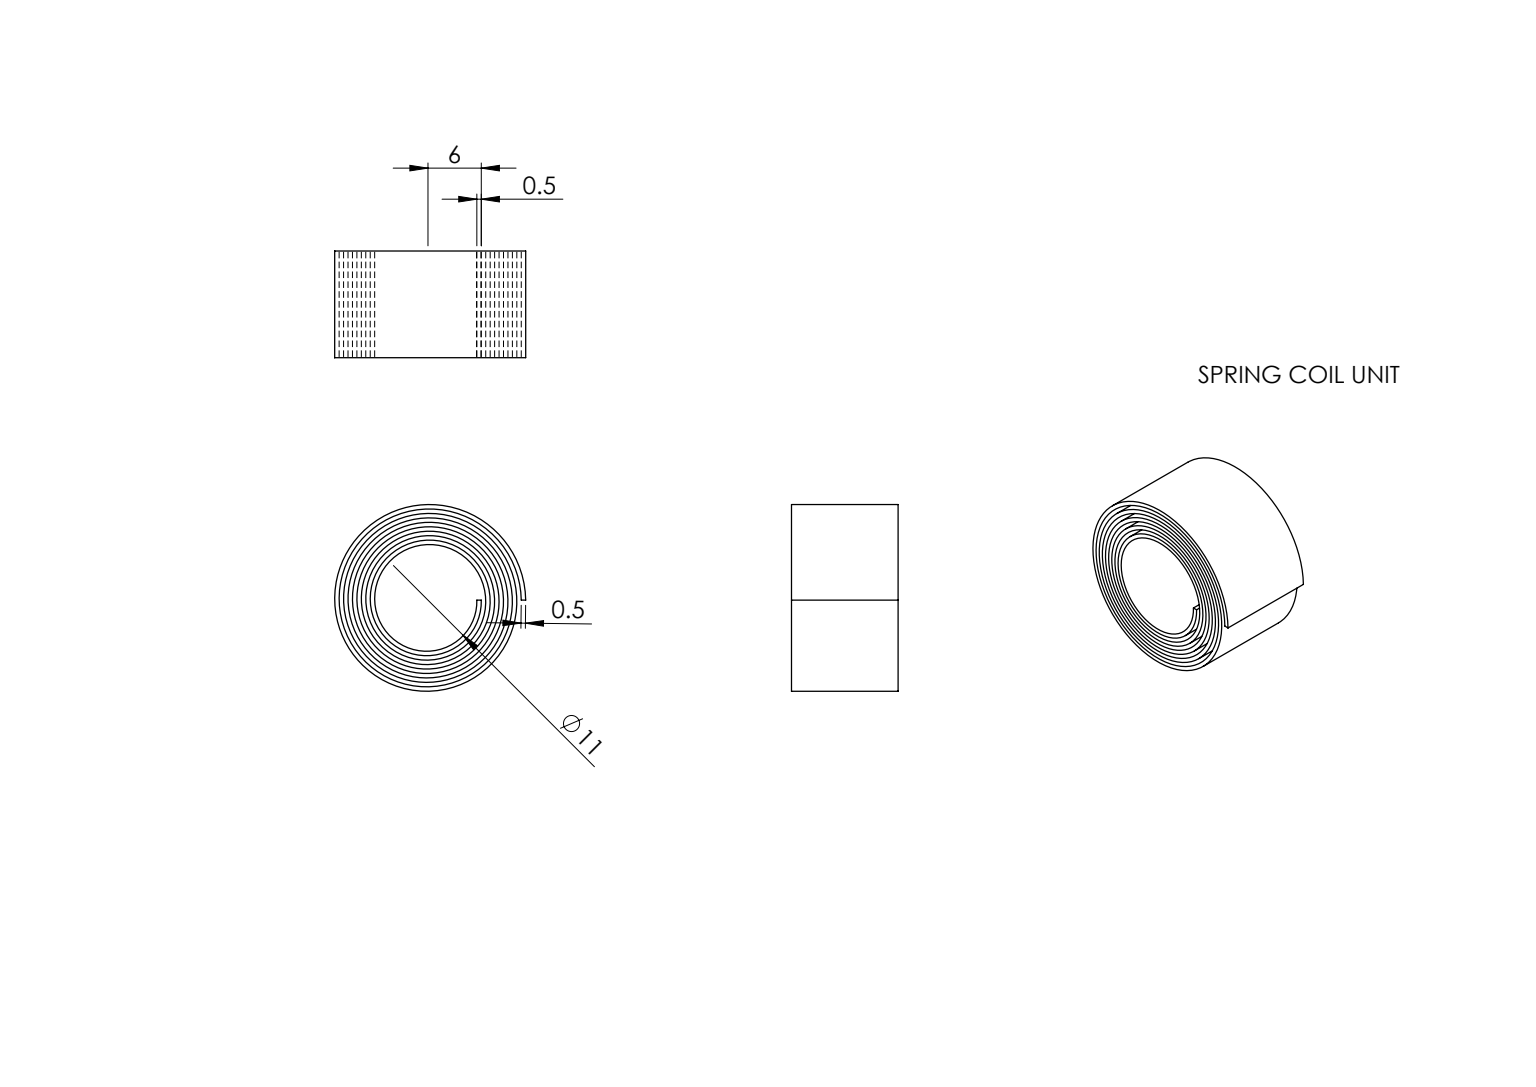
ISO-10303-21;
HEADER;
FILE_DESCRIPTION (('STEP AP214'),
    '1' );
FILE_NAME ('Spring Coil Unit.step',
    '2026-10-23T14:45:25',
    ( '' ),
    ( '' ),
    'SwSTEP 2.0',
    'SolidWorks 2026',
    '' );
FILE_SCHEMA (( 'AUTOMOTIVE_DESIGN' ));
ENDSEC;

DATA;
#1=CARTESIAN_POINT ( 'NONE',  ( -5.525185448606692695, 2.707100724334796649, 1.999999999999998224 ) ) ;
#7=CARTESIAN_POINT ( 'NONE',  ( 10.06493078320225010, 4.366638945734137245, 13.99999999999999645 ) ) ;
#13=CARTESIAN_POINT ( 'NONE',  ( 8.453438707197836521, 0.9797652757261499090, 14.00000000000000000 ) ) ;
#14=CARTESIAN_POINT ( 'NONE',  ( 3.892125705850321804, -6.036954802193386982, 1.999999999999998224 ) ) ;
#16=CARTESIAN_POINT ( 'NONE',  ( 7.990059919442007441, -3.149571442993018167, 14.00000000000000000 ) ) ;
#18=CARTESIAN_POINT ( 'NONE',  ( -2.440069559021881496, 10.46881825416662259, 1.999999999999998224 ) ) ;
#20=CARTESIAN_POINT ( 'NONE',  ( 5.887534416617372202, 3.663839002572494952, 13.99999999999999645 ) ) ;
#22=CARTESIAN_POINT ( 'NONE',  ( -2.415560149437878668, -8.486491385245608754, 1.999999999999998224 ) ) ;
#24=CARTESIAN_POINT ( 'NONE',  ( 2.877506500681688006, 7.288437455188073955, 1.999999999999998224 ) ) ;
#32=CARTESIAN_POINT ( 'NONE',  ( -10.48421140591525713, 1.206973991593908169, 13.99999999999999645 ) ) ;
#33=AXIS2_PLACEMENT_3D ( 'NONE', #3461, #5223, #4408 ) ;
#38=CARTESIAN_POINT ( 'NONE',  ( -0.2798806129217078498, -8.779921314117062892, 14.00000000000000000 ) ) ;
#39=CARTESIAN_POINT ( 'NONE',  ( 6.444084565535371567, 4.617298776321547393, 1.999999999999998224 ) ) ;
#42=CARTESIAN_POINT ( 'NONE',  ( -2.415560149437796511, -8.486491385245610530, 14.00000000000000000 ) ) ;
#45=CARTESIAN_POINT ( 'NONE',  ( 8.595497693523489247, -5.345940745659027549, 1.999999999999998224 ) ) ;
#46=CARTESIAN_POINT ( 'NONE',  ( -5.651290410005069376, 9.082320918485367045, 1.999999999999998224 ) ) ;
#47=( GEOMETRIC_REPRESENTATION_CONTEXT ( 3 ) GLOBAL_UNCERTAINTY_ASSIGNED_CONTEXT ( ( #114 ) ) GLOBAL_UNIT_ASSIGNED_CONTEXT ( ( #3594, #2760, #4052 ) ) REPRESENTATION_CONTEXT ( 'NONE', 'WORKASPACE' ) );
#48=CARTESIAN_POINT ( 'NONE',  ( -1.424809953814591523, 6.586142414399822620, 13.99999999999999645 ) ) ;
#49=CARTESIAN_POINT ( 'NONE',  ( 7.716263785693136867, -3.801003699432787375, 1.999999999999998224 ) ) ;
#51=CARTESIAN_POINT ( 'NONE',  ( 6.638644669766898154, 2.135480210976827387, 1.999999999999998224 ) ) ;
#61=CARTESIAN_POINT ( 'NONE',  ( -3.798941939731700579, -9.621416145859109648, 13.99999999999999645 ) ) ;
#66=CARTESIAN_POINT ( 'NONE',  ( -7.161907081466633684, 5.673982509929174967, 14.00000000000000000 ) ) ;
#67=CARTESIAN_POINT ( 'NONE',  ( 7.024953159363688471, -4.052930060063556716, 1.999999999999998224 ) ) ;
#70=CARTESIAN_POINT ( 'NONE',  ( -7.550296695603107899, -2.566425989403007257, 1.999999999999998224 ) ) ;
#71=CARTESIAN_POINT ( 'NONE',  ( 0.7514524083000287957, 9.263466152293682754, 14.00000000000000000 ) ) ;
#74=CARTESIAN_POINT ( 'NONE',  ( 9.807503887220748950, -2.283819133639664489, 1.999999999999998224 ) ) ;
#75=CARTESIAN_POINT ( 'NONE',  ( 6.160418207306094018, 1.983851483784787373, 14.00000000000000000 ) ) ;
#76=CARTESIAN_POINT ( 'NONE',  ( -7.091148812992124739, -4.571561645351811976, 13.99999999999999645 ) ) ;
#77=CARTESIAN_POINT ( 'NONE',  ( -8.026550172065741506, -2.724140490265046122, 13.99999999999999645 ) ) ;
#79=CARTESIAN_POINT ( 'NONE',  ( -4.424777426321968576, -7.679192617323552739, 1.999999999999998224 ) ) ;
#80=CARTESIAN_POINT ( 'NONE',  ( 5.887534416617370425, 3.663839002572738313, 1.999999999999998224 ) ) ;
#89=CARTESIAN_POINT ( 'NONE',  ( -8.483256258862985177, -6.077987531410205868, 13.99999999999999645 ) ) ;
#95=CARTESIAN_POINT ( 'NONE',  ( -6.708753103182797162, 7.642576097240647570, 14.00000000000000000 ) ) ;
#96=CARTESIAN_POINT ( 'NONE',  ( 7.409328306158467825, 2.927536720054290775, 1.999999999999998224 ) ) ;
#97=CARTESIAN_POINT ( 'NONE',  ( 5.612687125617794592, -6.603876269260512188, 1.999999999999998224 ) ) ;
#98=CARTESIAN_POINT ( 'NONE',  ( -6.185289998984974780, -6.402116997106622520, 14.00000000000000000 ) ) ;
#100=CARTESIAN_POINT ( 'NONE',  ( -0.7077576507783156501, 10.75210906117156995, 1.999999999999998224 ) ) ;
#102=CARTESIAN_POINT ( 'NONE',  ( 5.103689747953259470, 6.014827819656690444, 13.99999999999999645 ) ) ;
#103=CARTESIAN_POINT ( 'NONE',  ( -8.388197440585694054, -1.387539741535495974, 13.99999999999999645 ) ) ;
#104=CARTESIAN_POINT ( 'NONE',  ( 1.492118473828444536, -5.588909376072072277, 14.00000000000000000 ) ) ;
#106=CARTESIAN_POINT ( 'NONE',  ( -8.126042061586874254, 2.755650963504471473, 1.999999999999998224 ) ) ;
#108=CARTESIAN_POINT ( 'NONE',  ( -0.5497243705170606898, -6.763214047005217999, 1.999999999999998224 ) ) ;
#113=SURFACE_STYLE_FILL_AREA ( #890 ) ;
#114=UNCERTAINTY_MEASURE_WITH_UNIT (LENGTH_MEASURE( 1.000000000000000082E-05 ), #3594, 'distance_accuracy_value', 'NONE');
#115=CARTESIAN_POINT ( 'NONE',  ( 5.800093669798302543, -8.375184749302979625, 13.99999999999999645 ) ) ;
#119=CARTESIAN_POINT ( 'NONE',  ( -3.139313036748870189, 9.741172307225710369, 14.00000000000000000 ) ) ;
#120=CARTESIAN_POINT ( 'NONE',  ( -0.2539011084975961174, 7.766605221862830533, 1.999999999999998224 ) ) ;
#122=CARTESIAN_POINT ( 'NONE',  ( -8.763921109942213405, 2.343993041296470459, 1.999999999999998224 ) ) ;
#123=CARTESIAN_POINT ( 'NONE',  ( -7.559400777704423646, -6.425066744314204215, 14.00000000000000000 ) ) ;
#126=CARTESIAN_POINT ( 'NONE',  ( 7.631804465921431913, -6.689046765414639495, 1.999999999999998224 ) ) ;
#129=CARTESIAN_POINT ( 'NONE',  ( 0.5754137710878940437, 8.770917875152660415, 13.99999999999999645 ) ) ;
#131=CARTESIAN_POINT ( 'NONE',  ( -9.772156678340820690, -2.119544458102139206, 1.999999999999998224 ) ) ;
#133=CARTESIAN_POINT ( 'NONE',  ( 3.747087600548639763, -7.295897990121164689, 1.999999999999998224 ) ) ;
#137=CARTESIAN_POINT ( 'NONE',  ( -7.019651866617071079, -0.1200674265790944856, 1.999999999999998224 ) ) ;
#140=CARTESIAN_POINT ( 'NONE',  ( -3.597458971453999066, 6.226096630968013024, 1.999999999999998224 ) ) ;
#152=CARTESIAN_POINT ( 'NONE',  ( -9.772156678340820690, -2.119544458102511353, 14.00000000000000000 ) ) ;
#153=CARTESIAN_POINT ( 'NONE',  ( 7.344045208304290639, 5.086154276871864610, 1.999999999999998224 ) ) ;
#156=CARTESIAN_POINT ( 'NONE',  ( 4.415008247871750058, 7.106745273741266189, 1.999999999999998224 ) ) ;
#157=CARTESIAN_POINT ( 'NONE',  ( -4.983290658054754019, 7.721050520723660604, 14.00000000000000000 ) ) ;
#162=CARTESIAN_POINT ( 'NONE',  ( -5.390757458300978300, 6.793134358447313836, 13.99999999999999645 ) ) ;
#164=CARTESIAN_POINT ( 'NONE',  ( -0.6809175113353352904, 10.25113960786383771, 1.999999999999998224 ) ) ;
#166=CARTESIAN_POINT ( 'NONE',  ( 3.388254439433305176, -8.575817650944026482, 1.999999999999998224 ) ) ;
#170=CARTESIAN_POINT ( 'NONE',  ( -1.320393794063943416, 6.095439640211752774, 1.999999999999998224 ) ) ;
#172=CARTESIAN_POINT ( 'NONE',  ( -4.975175822334872322, 5.137265612443480123, 1.999999999999998224 ) ) ;
#178=LINE ( 'NONE', #3662, #4829 ) ;
#181=CARTESIAN_POINT ( 'NONE',  ( 0.7514524083000287957, 9.263466152293682754, 14.00000000000000000 ) ) ;
#182=CARTESIAN_POINT ( 'NONE',  ( 4.043470907200509501, 7.877814422643418801, 1.999999999999998224 ) ) ;
#183=CARTESIAN_POINT ( 'NONE',  ( -1.480145937554574020, 8.115026467928048604, 1.999999999999998224 ) ) ;
#184=CARTESIAN_POINT ( 'NONE',  ( 7.258279873954945671, -6.354128476750924293, 14.00000000000000000 ) ) ;
#188=CARTESIAN_POINT ( 'NONE',  ( 5.326024957120313985, -1.813589758486611858, 14.00000000000000000 ) ) ;
#189=CARTESIAN_POINT ( 'NONE',  ( -2.179108132477381332, -10.08557389312607278, 13.99999999999999645 ) ) ;
#191=CARTESIAN_POINT ( 'NONE',  ( 3.896371052708265559, -4.167854722423870228, 14.00000000000000000 ) ) ;
#193=CARTESIAN_POINT ( 'NONE',  ( -1.063411474431080306, -9.238278818534249481, 1.999999999999998224 ) ) ;
#195=CARTESIAN_POINT ( 'NONE',  ( -6.742266116715657454, -1.811900715329134215, 1.999999999999998224 ) ) ;
#197=ORIENTED_EDGE ( 'NONE', *, *, #3580, .T. ) ;
#198=CARTESIAN_POINT ( 'NONE',  ( -6.041022033915842471, 3.753782041846908779, 1.999999999999998224 ) ) ;
#200=CARTESIAN_POINT ( 'NONE',  ( -3.379911625893651017, -5.460782782531100388, 13.99999999999999645 ) ) ;
#208=CARTESIAN_POINT ( 'NONE',  ( -8.440272934376206848, 1.393994921405934173, 1.999999999999998224 ) ) ;
#209=CARTESIAN_POINT ( 'NONE',  ( 4.326322805050086373, -6.952463250691143237, 13.99999999999999645 ) ) ;
#210=CARTESIAN_POINT ( 'NONE',  ( -2.067895747887561697, -9.596367745172036834, 1.999999999999998224 ) ) ;
#216=CARTESIAN_POINT ( 'NONE',  ( -1.105557477332586691, -6.708264047591377732, 14.00000000000000000 ) ) ;
#217=CARTESIAN_POINT ( 'NONE',  ( -8.745075223331019387, 3.959260399367729111, 13.99999999999999645 ) ) ;
#218=CARTESIAN_POINT ( 'NONE',  ( -4.354965481614496703, -8.841480220787186539, 1.999999999999998224 ) ) ;
#221=CARTESIAN_POINT ( 'NONE',  ( -0.1359230501497094012, -8.279147739300480424, 1.999999999999998224 ) ) ;
#226=CARTESIAN_POINT ( 'NONE',  ( 2.227988792049259814, 5.923272706911028251, 1.999999999999998224 ) ) ;
#228=CARTESIAN_POINT ( 'NONE',  ( 3.520917041835318173, -6.848083076130971669, 1.999999999999998224 ) ) ;
#236=CARTESIAN_POINT ( 'NONE',  ( -0.1359230501497094012, -8.279147739300480424, 1.999999999999998224 ) ) ;
#237=CARTESIAN_POINT ( 'NONE',  ( -5.921118896519415919, 6.318058289644736369, 13.99999999999999645 ) ) ;
#243=CARTESIAN_POINT ( 'NONE',  ( 6.004028658818958419, -2.715480180205860794, 14.00000000000000000 ) ) ;
#244=CARTESIAN_POINT ( 'NONE',  ( 3.917689075872249571, 9.035181080458080771, 13.99999999999999645 ) ) ;
#245=CARTESIAN_POINT ( 'NONE',  ( -0.5497243705170608008, -6.763214047005219776, 14.00000000000000000 ) ) ;
#249=CARTESIAN_POINT ( 'NONE',  ( -10.48421140591450751, 1.206973991593908169, 1.999999999999998224 ) ) ;
#253=CARTESIAN_POINT ( 'NONE',  ( 6.680730669075649608, 3.301097878975988387, 1.999999999999998224 ) ) ;
#255=CARTESIAN_POINT ( 'NONE',  ( -5.416162817796314144, -4.301262981183148426, 1.999999999999998224 ) ) ;
#256=CARTESIAN_POINT ( 'NONE',  ( -2.466819000628106551, 6.242838961510105200, 1.999999999999998224 ) ) ;
#258=CARTESIAN_POINT ( 'NONE',  ( 4.793600759081160234, 4.956424179878266223, 13.99999999999999645 ) ) ;
#261=VERTEX_POINT ( 'NONE', #4126 ) ;
#264=CARTESIAN_POINT ( 'NONE',  ( 3.747087600548639763, -7.295897990121164689, 1.999999999999998224 ) ) ;
#265=CARTESIAN_POINT ( 'NONE',  ( -7.364573508975984062, 1.714675912027187943, 13.99999999999999645 ) ) ;
#266=CARTESIAN_POINT ( 'NONE',  ( 5.030817567586885808, 9.062633982223131213, 14.00000000000000000 ) ) ;
#269=PRODUCT_DEFINITION_SHAPE ( 'NONE', 'NONE',  #3907 ) ;
#273=CARTESIAN_POINT ( 'NONE',  ( -2.717942380035140992, -6.274577315194989957, 14.00000000000000000 ) ) ;
#274=CARTESIAN_POINT ( 'NONE',  ( -1.592064345877354903, 9.625584969239746158, 13.99999999999999645 ) ) ;
#275=CARTESIAN_POINT ( 'NONE',  ( 4.290186206382709422, 5.996800006796702220, 14.00000000000000000 ) ) ;
#277=CARTESIAN_POINT ( 'NONE',  ( 7.631804465921431913, -6.689046765414639495, 1.999999999999998224 ) ) ;
#280=CARTESIAN_POINT ( 'NONE',  ( -7.652305818843809782, 2.590529227167489790, 1.999999999999998224 ) ) ;
#282=CARTESIAN_POINT ( 'NONE',  ( -1.189470317277863565, -7.202885406307538041, 13.99999999999999645 ) ) ;
#283=CARTESIAN_POINT ( 'NONE',  ( 0.000000000000000000, 0.000000000000000000, 0.000000000000000000 ) ) ;
#289=CARTESIAN_POINT ( 'NONE',  ( -8.017392084630253990, -4.988806607527433989, 1.999999999999998224 ) ) ;
#290=CARTESIAN_POINT ( 'NONE',  ( 8.697835924490034287, 4.836984431370582982, 13.99999999999999645 ) ) ;
#291=CARTESIAN_POINT ( 'NONE',  ( 9.925004466819306259, 3.374327561486830440, 14.00000000000000000 ) ) ;
#296=CARTESIAN_POINT ( 'NONE',  ( -5.034899347480884302, -4.722558430572732391, 14.00000000000000000 ) ) ;
#297=CARTESIAN_POINT ( 'NONE',  ( 5.099673838353210975, -8.834479793763010846, 13.99999999999999645 ) ) ;
#299=CARTESIAN_POINT ( 'NONE',  ( 7.439669587982604249, 0.9822684312230363091, 14.00000000000000000 ) ) ;
#301=CARTESIAN_POINT ( 'NONE',  ( -8.017392084630253990, -4.988806607527433989, 1.999999999999998224 ) ) ;
#305=CARTESIAN_POINT ( 'NONE',  ( 6.929006764466009827, 4.804313515625705300, 1.999999999999998224 ) ) ;
#307=CARTESIAN_POINT ( 'NONE',  ( 4.243312049792013596, -4.537448458213932945, 1.999999999999998224 ) ) ;
#308=CARTESIAN_POINT ( 'NONE',  ( -7.375360291558942905, -1.341686286798741357, 13.99999999999999645 ) ) ;
#311=CARTESIAN_POINT ( 'NONE',  ( -4.354965481614496703, -8.841480220787186539, 1.999999999999998224 ) ) ;
#320=CARTESIAN_POINT ( 'NONE',  ( 6.971023843911450690, -5.915260676233724091, 13.99999999999999645 ) ) ;
#321=CARTESIAN_POINT ( 'NONE',  ( 8.774740126074163982, 5.663528079765788981, 14.00000000000000000 ) ) ;
#327=CARTESIAN_POINT ( 'NONE',  ( -6.334648143026945455, -2.872559841354017429, 14.00000000000000000 ) ) ;
#329=CARTESIAN_POINT ( 'NONE',  ( 10.40193138080327628, 3.529992181067589829, 13.99999999999999645 ) ) ;
#332=CARTESIAN_POINT ( 'NONE',  ( 4.443413384189735638, 4.597174039215665253, 14.00000000000000000 ) ) ;
#335=CARTESIAN_POINT ( 'NONE',  ( 9.807503887220748950, -2.283819133639664489, 1.999999999999998224 ) ) ;
#339=CARTESIAN_POINT ( 'NONE',  ( 6.037635170864973588, 5.848285684830694997, 1.999999999999998224 ) ) ;
#343=CARTESIAN_POINT ( 'NONE',  ( 6.997680802075244344, 0.4609939245309428446, 13.99999999999999645 ) ) ;
#344=CARTESIAN_POINT ( 'NONE',  ( -9.772156678340820690, -2.119544458102139206, 1.999999999999998224 ) ) ;
#351=CARTESIAN_POINT ( 'NONE',  ( 2.701324588234351953, 8.405562337868641265, 13.99999999999999645 ) ) ;
#358=CARTESIAN_POINT ( 'NONE',  ( 8.156937663706065322, 2.333191796391004047, 14.00000000000000000 ) ) ;
#359=CARTESIAN_POINT ( 'NONE',  ( -7.945634105012030268, -6.745245841439798440, 13.99999999999999645 ) ) ;
#361=CARTESIAN_POINT ( 'NONE',  ( 6.523553822664519330, -0.1051741892335816969, 14.00000000000000000 ) ) ;
#363=CARTESIAN_POINT ( 'NONE',  ( -4.581738566658409617, -9.288989786611782762, 1.999999999999998224 ) ) ;
#365=CARTESIAN_POINT ( 'NONE',  ( -5.623512120026317618, -3.262381593763366450, 13.99999999999999645 ) ) ;
#366=CARTESIAN_POINT ( 'NONE',  ( 7.097632634466812362, -2.668286824979932970, 1.999999999999998224 ) ) ;
#368=CARTESIAN_POINT ( 'NONE',  ( 5.586635445632386343, -4.430858740432560339, 13.99999999999999645 ) ) ;
#369=CARTESIAN_POINT ( 'NONE',  ( -8.332455577110955858, 5.761155596213678010, 1.999999999999998224 ) ) ;
#375=CARTESIAN_POINT ( 'NONE',  ( -0.7976699882156008670, 9.736979168371714621, 13.99999999999999645 ) ) ;
#376=PLANE ( 'NONE',  #33 ) ;
#381=CARTESIAN_POINT ( 'NONE',  ( -7.550296695602809471, -2.566425989403007257, 14.00000000000000000 ) ) ;
#382=CARTESIAN_POINT ( 'NONE',  ( 1.869626052002579808, 6.555486721476420087, 1.999999999999998224 ) ) ;
#386=CARTESIAN_POINT ( 'NONE',  ( -6.453089103408906624, 4.947336467533685500, 14.00000000000000000 ) ) ;
#390=CARTESIAN_POINT ( 'NONE',  ( 5.213743241621229707, -4.883528188333805531, 13.99999999999999645 ) ) ;
#392=CARTESIAN_POINT ( 'NONE',  ( -8.999716648909558359, -0.5976852874978595409, 1.999999999999998224 ) ) ;
#393=CARTESIAN_POINT ( 'NONE',  ( 5.103689747953258582, 6.014827819656408892, 1.999999999999998224 ) ) ;
#394=CARTESIAN_POINT ( 'NONE',  ( 7.024953159363689359, -4.052930060063556716, 13.99999999999999645 ) ) ;
#397=( LENGTH_UNIT ( ) NAMED_UNIT ( * ) SI_UNIT ( .MILLI., .METRE. ) );
#399=CARTESIAN_POINT ( 'NONE',  ( -8.072272399572318236, -5.790267008923112080, 1.999999999999998224 ) ) ;
#406=CARTESIAN_POINT ( 'NONE',  ( 8.640499015841685448, 2.466831329604985079, 13.99999999999999645 ) ) ;
#415=CARTESIAN_POINT ( 'NONE',  ( 5.528193227149303723, 6.314447692498919018, 14.00000000000000000 ) ) ;
#416=CARTESIAN_POINT ( 'NONE',  ( -9.197478219253614640, 5.306711421960436326, 13.99999999999999645 ) ) ;
#419=CARTESIAN_POINT ( 'NONE',  ( 1.760389272475214373, -7.536528230137969686, 14.00000000000000000 ) ) ;
#423=CARTESIAN_POINT ( 'NONE',  ( -3.379911625893651017, -5.460782782531100388, 13.99999999999999645 ) ) ;
#425=CARTESIAN_POINT ( 'NONE',  ( -6.700137237869126849, -5.881230172875862472, 1.999999999999998224 ) ) ;
#427=ORIENTED_EDGE ( 'NONE', *, *, #2908, .T. ) ;
#428=CARTESIAN_POINT ( 'NONE',  ( -5.402835942920797940, -5.063607225391133504, 1.999999999999998224 ) ) ;
#439=CARTESIAN_POINT ( 'NONE',  ( -7.945634105012030268, -6.745245841439798440, 13.99999999999999645 ) ) ;
#440=ORIENTED_EDGE ( 'NONE', *, *, #5176, .T. ) ;
#444=CARTESIAN_POINT ( 'NONE',  ( -8.547479018125100581, -2.754496926847988636, 14.00000000000000000 ) ) ;
#445=CARTESIAN_POINT ( 'NONE',  ( -3.379911625893426308, -5.460782782531098611, 1.999999999999998224 ) ) ;
#448=CARTESIAN_POINT ( 'NONE',  ( 2.369394374793903246, -7.353877281245580377, 14.00000000000000000 ) ) ;
#450=CARTESIAN_POINT ( 'NONE',  ( 10.86297249782008123, 1.796588950249126349, 1.999999999999998224 ) ) ;
#451=CARTESIAN_POINT ( 'NONE',  ( 6.804422688527093754, 1.586354726854036112, 13.99999999999999645 ) ) ;
#453=CARTESIAN_POINT ( 'NONE',  ( -1.001529162299556797, -8.740421795711002417, 1.999999999999998224 ) ) ;
#454=CARTESIAN_POINT ( 'NONE',  ( 6.460119401626724489, -2.924461030940388895, 1.999999999999998224 ) ) ;
#456=SURFACE_SIDE_STYLE ('',( #113 ) ) ;
#458=CARTESIAN_POINT ( 'NONE',  ( 3.622712361020122618, 5.236663886535374957, 1.999999999999998224 ) ) ;
#462=CARTESIAN_POINT ( 'NONE',  ( -8.741731599017841248, 6.051300285686072478, 13.99999999999999645 ) ) ;
#467=CARTESIAN_POINT ( 'NONE',  ( -6.453089103408906624, 4.947336467533685500, 14.00000000000000000 ) ) ;
#468=CARTESIAN_POINT ( 'NONE',  ( 2.877506500681688006, 7.288437455188073955, 1.999999999999998224 ) ) ;
#469=DIRECTION ( 'NONE',  ( 0.000000000000000000, -0.000000000000000000, 1.000000000000000000 ) ) ;
#470=CARTESIAN_POINT ( 'NONE',  ( 7.311638624438943523, 4.225618826270838291, 14.00000000000000000 ) ) ;
#472=CARTESIAN_POINT ( 'NONE',  ( -6.726831604608804582, -7.927219868180728213, 1.999999999999998224 ) ) ;
#476=CARTESIAN_POINT ( 'NONE',  ( 3.433597602020624251, -9.098706718023301221, 1.999999999999998224 ) ) ;
#478=CARTESIAN_POINT ( 'NONE',  ( -7.227555219266156072, -1.939125212622417660, 1.999999999999998224 ) ) ;
#482=CARTESIAN_POINT ( 'NONE',  ( 2.389076732465379216, -5.237771676861643577, 1.999999999999998224 ) ) ;
#483=CARTESIAN_POINT ( 'NONE',  ( -5.021280548121167975, 3.603657539922314967, 2.000000000001176392 ) ) ;
#487=CARTESIAN_POINT ( 'NONE',  ( 2.803319092186594474, 10.45862564946370021, 13.99999999999999645 ) ) ;
#494=CARTESIAN_POINT ( 'NONE',  ( 3.713512749563263604, 8.576920285551967282, 14.00000000000000000 ) ) ;
#495=CARTESIAN_POINT ( 'NONE',  ( 7.761517335261689965, -2.213789340049559407, 1.999999999999998224 ) ) ;
#497=CARTESIAN_POINT ( 'NONE',  ( -6.453089103408601090, 4.947336467533990145, 1.999999999999998224 ) ) ;
#498=CARTESIAN_POINT ( 'NONE',  ( -3.391372024942433949, 7.476497417048839189, 14.00000000000000000 ) ) ;
#502=CARTESIAN_POINT ( 'NONE',  ( 9.077580196902394150, 4.112174628513753483, 1.999999999999998224 ) ) ;
#503=CARTESIAN_POINT ( 'NONE',  ( -2.283612537812034216, 5.775797914528924437, 14.00000000000000000 ) ) ;
#504=CARTESIAN_POINT ( 'NONE',  ( -8.026550172065741506, -2.724140490265046122, 13.99999999999999645 ) ) ;
#506=CARTESIAN_POINT ( 'NONE',  ( 2.877506500681688895, 7.288437455188075731, 13.99999999999999645 ) ) ;
#508=CARTESIAN_POINT ( 'NONE',  ( -9.031632682309719939, 0.1436733667526190195, 1.999999999999998224 ) ) ;
#510=CLOSED_SHELL ( 'NONE', ( #4640, #572, #825, #4442, #4161, #3825 ) ) ;
#511=VECTOR ( 'NONE', #2427, 1000.000000000000000 ) ;
#512=CARTESIAN_POINT ( 'NONE',  ( 7.937472058416057408, 1.044590838406009414, 1.999999999999998224 ) ) ;
#513=CARTESIAN_POINT ( 'NONE',  ( 6.000000000000000000, 0.000000000000000000, 1.999999999999998224 ) ) ;
#518=CARTESIAN_POINT ( 'NONE',  ( -3.595699629853521984, 5.016010494498948091, 1.999999999999998224 ) ) ;
#527=CARTESIAN_POINT ( 'NONE',  ( -8.765969750978372943, 5.050798838973364902, 14.00000000000000000 ) ) ;
#528=CARTESIAN_POINT ( 'NONE',  ( -0.8890388043606449742, 7.706404363472288743, 1.999999999999998224 ) ) ;
#531=CARTESIAN_POINT ( 'NONE',  ( -5.048038583874033591, -7.300734008993713609, 1.999999999999998224 ) ) ;
#532=CARTESIAN_POINT ( 'NONE',  ( -6.398096652174581678, -7.548242073784473760, 14.00000000000000000 ) ) ;
#535=CARTESIAN_POINT ( 'NONE',  ( -3.287100391418392942, 10.22059872437900019, 1.999999999999998224 ) ) ;
#536=CARTESIAN_POINT ( 'NONE',  ( 3.896371052708265559, -4.167854722423870228, 14.00000000000000000 ) ) ;
#537=CARTESIAN_POINT ( 'NONE',  ( -5.210352092881700869, -6.569156856910654874, 13.99999999999999645 ) ) ;
#538=CARTESIAN_POINT ( 'NONE',  ( 3.747087600548785868, -7.295897990121166465, 13.99999999999999645 ) ) ;
#539=CARTESIAN_POINT ( 'NONE',  ( -6.069783318623454882, -0.2142533344233820691, 14.00000000000000000 ) ) ;
#540=CARTESIAN_POINT ( 'NONE',  ( -2.153669193480073574, -8.035861145135083206, 1.999999999999998224 ) ) ;
#548=CARTESIAN_POINT ( 'NONE',  ( -5.651290410005071152, 9.082320918485368821, 13.99999999999999645 ) ) ;
#550=CARTESIAN_POINT ( 'NONE',  ( 6.000000000000000000, 0.000000000000000000, 1.999999999999998224 ) ) ;
#553=CARTESIAN_POINT ( 'NONE',  ( -5.592500163774714039, 7.275211197852027745, 14.00000000000000000 ) ) ;
#554=CARTESIAN_POINT ( 'NONE',  ( 7.025143070632193343, -0.1151745751371896220, 1.999999999999998224 ) ) ;
#555=CARTESIAN_POINT ( 'NONE',  ( -9.031632682309719939, 0.1436733667526190195, 1.999999999999998224 ) ) ;
#556=CARTESIAN_POINT ( 'NONE',  ( -2.067895747887562141, -9.596367745172036834, 14.00000000000000000 ) ) ;
#558=CARTESIAN_POINT ( 'NONE',  ( -7.035243215357268376, 8.023489478516459883, 1.999999999999998224 ) ) ;
#560=CARTESIAN_POINT ( 'NONE',  ( 5.500000000000001776, 0.000000000000000000, 14.00000000000000000 ) ) ;
#561=CARTESIAN_POINT ( 'NONE',  ( 0.5432484998931954578, -8.249156888542636068, 13.99999999999999645 ) ) ;
#562=CARTESIAN_POINT ( 'NONE',  ( 5.526041665711820983, -0.8982374663919268087, 14.00000000000000000 ) ) ;
#564=CARTESIAN_POINT ( 'NONE',  ( -8.026550172065139321, -2.724140490265046122, 1.999999999999998224 ) ) ;
#566=CARTESIAN_POINT ( 'NONE',  ( 2.161943361801394570, -6.363123982928429179, 1.999999999999998224 ) ) ;
#568=CARTESIAN_POINT ( 'NONE',  ( 4.848934754808810865, -4.539135254905419359, 1.999999999999998224 ) ) ;
#570=EDGE_CURVE ( 'NONE', #3843, #2002, #3145, .T. ) ;
#571=CARTESIAN_POINT ( 'NONE',  ( -6.576488680450180979, -0.2289623203888878078, 13.99999999999999645 ) ) ;
#572=ADVANCED_FACE ( 'NONE', ( #4032 ), #4002, .T. ) ;
#580=CARTESIAN_POINT ( 'NONE',  ( -9.031632682309723492, 0.1436733667526614300, 14.00000000000000000 ) ) ;
#581=CARTESIAN_POINT ( 'NONE',  ( -6.465640026559585252, 4.020973141381892546, 1.999999999999998224 ) ) ;
#583=CARTESIAN_POINT ( 'NONE',  ( 7.925371078819430259, 2.990572132494937474, 1.999999999999998224 ) ) ;
#584=CARTESIAN_POINT ( 'NONE',  ( -8.757712506721391676, -2.046213373001789737, 14.00000000000000000 ) ) ;
#587=CARTESIAN_POINT ( 'NONE',  ( 11.00000000000000355, -2.485533480423018915E-14, 1.999999999999998224 ) ) ;
#589=CARTESIAN_POINT ( 'NONE',  ( -5.525185448606695360, 2.707100724334913444, 14.00000000000000000 ) ) ;
#590=CARTESIAN_POINT ( 'NONE',  ( 8.454926800553035804, -3.338224220245739726, 13.99999999999999645 ) ) ;
#592=CARTESIAN_POINT ( 'NONE',  ( -5.748891254250207083, -8.037420881456807109, 1.999999999999998224 ) ) ;
#594=CARTESIAN_POINT ( 'NONE',  ( 8.396466517619506575, 3.163083589105210258, 1.999999999999998224 ) ) ;
#600=CARTESIAN_POINT ( 'NONE',  ( -1.105557477332586247, -6.708264047591375956, 1.999999999999998224 ) ) ;
#603=CARTESIAN_POINT ( 'NONE',  ( -2.189112655477410740, -6.464091385745793339, 1.999999999999998224 ) ) ;
#611=CARTESIAN_POINT ( 'NONE',  ( -0.7616497023963333390, 9.236585841461440793, 14.00000000000000000 ) ) ;
#613=CARTESIAN_POINT ( 'NONE',  ( -5.390757458300977412, 6.793134358447004750, 1.999999999999998224 ) ) ;
#615=CARTESIAN_POINT ( 'NONE',  ( -7.986673696634112751, -0.6581801297105769333, 1.999999999999998224 ) ) ;
#616=CARTESIAN_POINT ( 'NONE',  ( 8.549805251451807919, -4.382211019330642721, 14.00000000000000000 ) ) ;
#621=CARTESIAN_POINT ( 'NONE',  ( -5.021280548128706833, 3.603657539914777885, 14.00000000000094147 ) ) ;
#623=CARTESIAN_POINT ( 'NONE',  ( 0.3355163285737458034, -10.27362971114551371, 13.99999999999999645 ) ) ;
#626=CARTESIAN_POINT ( 'NONE',  ( 2.667884741302309237, 9.975564253400264647, 1.999999999999998224 ) ) ;
#628=CARTESIAN_POINT ( 'NONE',  ( 4.683456943470878819, 7.530568860026273015, 1.999999999999998224 ) ) ;
#631=CARTESIAN_POINT ( 'NONE',  ( 6.160418207306092242, 1.983851483784910164, 1.999999999999998224 ) ) ;
#633=CARTESIAN_POINT ( 'NONE',  ( 1.540339863274624577, 7.144097608501353669, 1.999999999999998224 ) ) ;
#635=CARTESIAN_POINT ( 'NONE',  ( 1.623707939105870413, -6.078451570951948213, 13.99999999999999645 ) ) ;
#642=CARTESIAN_POINT ( 'NONE',  ( 10.36702220812670028, 1.720931399333114120, 14.00000000000000000 ) ) ;
#643=CARTESIAN_POINT ( 'NONE',  ( 8.164254108709977586, -4.026826083952141033, 1.999999999999998224 ) ) ;
#644=CARTESIAN_POINT ( 'NONE',  ( -7.763712483375483586, -3.368527140561099031, 13.99999999999999645 ) ) ;
#645=CARTESIAN_POINT ( 'NONE',  ( -1.271096247112533995, -9.720655361064800104, 1.999999999999998224 ) ) ;
#646=CARTESIAN_POINT ( 'NONE',  ( 9.320190601378300244, -2.164585516638619200, 14.00000000000000000 ) ) ;
#650=CARTESIAN_POINT ( 'NONE',  ( 6.340368144647111848, -1.697206311171021831, 14.00000000000000000 ) ) ;
#651=CARTESIAN_POINT ( 'NONE',  ( -9.026614039607444795, -2.903226997913483487, 13.99999999999999645 ) ) ;
#654=CARTESIAN_POINT ( 'NONE',  ( -4.668631340267960894, 9.078485505801564770, 1.999999999999998224 ) ) ;
#656=CARTESIAN_POINT ( 'NONE',  ( 7.748217264256983761, 4.472783157626249562, 1.999999999999998224 ) ) ;
#659=CARTESIAN_POINT ( 'NONE',  ( -3.597458971453999066, 6.226096630968013024, 1.999999999999998224 ) ) ;
#660=VERTEX_POINT ( 'NONE', #4381 ) ;
#661=CARTESIAN_POINT ( 'NONE',  ( 6.268835244667307904, -4.335177162149147279, 1.999999999999998224 ) ) ;
#663=FACE_OUTER_BOUND ( 'NONE', #2351, .T. ) ;
#666=DIRECTION ( 'NONE',  ( -1.000000000000000000, -0.000000000000000000, -0.000000000000000000 ) ) ;
#670=CARTESIAN_POINT ( 'NONE',  ( -1.063411474431080306, -9.238278818534249481, 1.999999999999998224 ) ) ;
#671=CARTESIAN_POINT ( 'NONE',  ( -6.848710654519975627, 5.255840572796830479, 13.99999999999999645 ) ) ;
#677=CARTESIAN_POINT ( 'NONE',  ( -4.975175822334874098, 5.137265612443751017, 14.00000000000000000 ) ) ;
#678=CARTESIAN_POINT ( 'NONE',  ( -6.537688394901546296, -6.759197365499824528, 13.99999999999999645 ) ) ;
#680=CARTESIAN_POINT ( 'NONE',  ( -6.876639332705559937, 1.598006320995821516, 14.00000000000000000 ) ) ;
#683=CARTESIAN_POINT ( 'NONE',  ( -10.42442484909470046, -1.371544430045556373, 1.999999999999998224 ) ) ;
#688=CARTESIAN_POINT ( 'NONE',  ( 4.064490656457592443, -6.524520197619557926, 1.999999999999998224 ) ) ;
#690=CARTESIAN_POINT ( 'NONE',  ( 6.496939485553420823, 0.4301729194711073623, 1.999999999999998224 ) ) ;
#692=CARTESIAN_POINT ( 'NONE',  ( -3.886954398759499885, 5.424498719065524277, 1.999999999999998224 ) ) ;
#693=CARTESIAN_POINT ( 'NONE',  ( 7.025143070632195119, -0.1151745751371588272, 13.99999999999999645 ) ) ;
#704=CARTESIAN_POINT ( 'NONE',  ( -2.263950162103713915, 8.438937471999857109, 1.999999999999998224 ) ) ;
#705=CARTESIAN_POINT ( 'NONE',  ( -4.372214883940321428, 6.312905667202753257, 13.99999999999999645 ) ) ;
#713=CARTESIAN_POINT ( 'NONE',  ( 6.496939485553422600, 0.4301729194711386151, 14.00000000000000000 ) ) ;
#714=CARTESIAN_POINT ( 'NONE',  ( 0.7976699882155482424, 9.763020831628288931, 13.99999999999999645 ) ) ;
#716=CARTESIAN_POINT ( 'NONE',  ( 4.848934754808812642, -4.539135254905673378, 14.00000000000000000 ) ) ;
#719=CARTESIAN_POINT ( 'NONE',  ( 10.02239396097947655, -0.6576683464576721372, 1.999999999999998224 ) ) ;
#722=CARTESIAN_POINT ( 'NONE',  ( -1.480145937554574020, 8.115026467928048604, 1.999999999999998224 ) ) ;
#724=CARTESIAN_POINT ( 'NONE',  ( 4.366464973618273682, -5.686602709308030690, 13.99999999999999645 ) ) ;
#729=CARTESIAN_POINT ( 'NONE',  ( -0.1462562576243746360, 8.775315755191545719, 1.999999999999998224 ) ) ;
#730=CARTESIAN_POINT ( 'NONE',  ( 7.422282976138728117, -5.315384720684047437, 13.99999999999999645 ) ) ;
#736=CARTESIAN_POINT ( 'NONE',  ( 3.621982275015807939, -5.614208739972780471, 14.00000000000000000 ) ) ;
#737=CARTESIAN_POINT ( 'NONE',  ( -1.063411474431080528, -9.238278818535565762, 13.99999999999999645 ) ) ;
#738=CARTESIAN_POINT ( 'NONE',  ( -4.184906021401652687, -5.457255036755483069, 14.00000000000000000 ) ) ;
#740=CARTESIAN_POINT ( 'NONE',  ( 5.800093669797941054, -8.375184749302256648, 1.999999999999998224 ) ) ;
#743=CARTESIAN_POINT ( 'NONE',  ( 3.810368753942602993, 7.433568398487427231, 1.999999999999998224 ) ) ;
#745=CARTESIAN_POINT ( 'NONE',  ( -2.352725117874390648, -6.938351456669185069, 13.99999999999999645 ) ) ;
#747=CARTESIAN_POINT ( 'NONE',  ( -7.304208470130000741, 7.056621303511527721, 1.999999999999998224 ) ) ;
#755=CARTESIAN_POINT ( 'NONE',  ( 8.454926800553035804, -3.338224220245739726, 13.99999999999999645 ) ) ;
#762=CARTESIAN_POINT ( 'NONE',  ( -0.5497243705170608008, -6.763214047005219776, 14.00000000000000000 ) ) ;
#763=CARTESIAN_POINT ( 'NONE',  ( -6.726831604608805470, -7.927219868181097695, 13.99999999999999645 ) ) ;
#765=CARTESIAN_POINT ( 'NONE',  ( 2.227988792049260702, 5.923272706910787555, 14.00000000000000000 ) ) ;
#767=CARTESIAN_POINT ( 'NONE',  ( -1.342170334697201595, -10.21728332006300199, 1.999999999999998224 ) ) ;
#771=CARTESIAN_POINT ( 'NONE',  ( -3.987536574860945038, 7.161134007378406885, 1.999999999999998224 ) ) ;
#773=CARTESIAN_POINT ( 'NONE',  ( -4.310533329765174670, 5.077046166955135220, 13.99999999999952927 ) ) ;
#776=CARTESIAN_POINT ( 'NONE',  ( 2.992331685656917539, 8.840389773664522721, 1.999999999999998224 ) ) ;
#783=CARTESIAN_POINT ( 'NONE',  ( -9.533152408061619454, 0.1566715252476607312, 13.99999999999999645 ) ) ;
#791=CARTESIAN_POINT ( 'NONE',  ( -0.1241967792452473573, -7.777596356722547455, 14.00000000000000000 ) ) ;
#792=CARTESIAN_POINT ( 'NONE',  ( -0.8811140424828312057, 6.693995663234410642, 1.999999999999998224 ) ) ;
#796=CARTESIAN_POINT ( 'NONE',  ( -6.742266116715659230, -1.811900715328871092, 14.00000000000000000 ) ) ;
#799=CARTESIAN_POINT ( 'NONE',  ( -3.290073422422500560, -8.739709727800574868, 1.999999999999998224 ) ) ;
#803=CARTESIAN_POINT ( 'NONE',  ( 8.477027301005913174, -1.108685663976167080, 1.999999999999998224 ) ) ;
#806=CARTESIAN_POINT ( 'NONE',  ( 0.5931392160223177834, -7.236979168992432321, 13.99999999999999645 ) ) ;
#807=CARTESIAN_POINT ( 'NONE',  ( 9.348788865897812883, 1.705571004836294646, 1.999999999999998224 ) ) ;
#814=CARTESIAN_POINT ( 'NONE',  ( -8.402144917908875854, 4.670158400850172420, 13.99999999999999645 ) ) ;
#820=CARTESIAN_POINT ( 'NONE',  ( 6.591354251721611490, -5.587324598951901145, 14.00000000000000000 ) ) ;
#821=CARTESIAN_POINT ( 'NONE',  ( -6.112420884766618379, -2.295018720694776526, 1.999999999999998224 ) ) ;
#824=CARTESIAN_POINT ( 'NONE',  ( -6.281085993838468440, -4.827840781183066809, 14.00000000000000000 ) ) ;
#825=ADVANCED_FACE ( 'NONE', ( #663 ), #4177, .F. ) ;
#827=CARTESIAN_POINT ( 'NONE',  ( -7.035243215357268376, 8.023489478516459883, 1.999999999999998224 ) ) ;
#828=CARTESIAN_POINT ( 'NONE',  ( -4.492165532403490147, -5.853844512260857336, 13.99999999999999645 ) ) ;
#830=CARTESIAN_POINT ( 'NONE',  ( -2.970508497641843881, 8.737606122598624125, 1.999999999999998224 ) ) ;
#831=CARTESIAN_POINT ( 'NONE',  ( 4.585040342817966241, 6.402697129001492904, 1.999999999999998224 ) ) ;
#832=CARTESIAN_POINT ( 'NONE',  ( 7.748217264258252968, 4.472783157626409434, 13.99999999999999645 ) ) ;
#835=CARTESIAN_POINT ( 'NONE',  ( 8.549805251451806143, -4.382211019330641832, 1.999999999999998224 ) ) ;
#839=CARTESIAN_POINT ( 'NONE',  ( 1.999247522871012483, 8.586038698135613600, 13.99999999999999645 ) ) ;
#845=CARTESIAN_POINT ( 'NONE',  ( -3.813875884798381577, -6.869235835554827752, 14.00000000000000000 ) ) ;
#846=CARTESIAN_POINT ( 'NONE',  ( -5.978927507574433697, 2.933119789328457294, 1.999999999999998224 ) ) ;
#849=CARTESIAN_POINT ( 'NONE',  ( 8.477027301005275461, -1.108685663976147318, 14.00000000000000000 ) ) ;
#852=CARTESIAN_POINT ( 'NONE',  ( 11.00000000000000355, -2.485533480423018915E-14, 1.999999999999998224 ) ) ;
#854=CARTESIAN_POINT ( 'NONE',  ( -3.886954398759500773, 5.424498719065526053, 13.99999999999999645 ) ) ;
#856=CARTESIAN_POINT ( 'NONE',  ( 9.164356920907600568, 2.464151434936005192, 1.999999999999998224 ) ) ;
#857=CARTESIAN_POINT ( 'NONE',  ( -3.989331152809321157, -6.191695749071041810, 1.999999999999998224 ) ) ;
#858=CARTESIAN_POINT ( 'NONE',  ( 6.444084565535373343, 4.617298776321548281, 13.99999999999999645 ) ) ;
#865=ORIENTED_EDGE ( 'NONE', *, *, #2172, .F. ) ;
#868=CARTESIAN_POINT ( 'NONE',  ( 0.3355163285737458034, -10.27362971114551371, 13.99999999999999645 ) ) ;
#875=CARTESIAN_POINT ( 'NONE',  ( -7.588772809867895930, -4.728083520431684228, 14.00000000000000000 ) ) ;
#876=CARTESIAN_POINT ( 'NONE',  ( -8.483256258862985177, -6.077987531410205868, 13.99999999999999645 ) ) ;
#879=CARTESIAN_POINT ( 'NONE',  ( 6.268835244667308793, -4.335177162149436825, 14.00000000000000000 ) ) ;
#883=CARTESIAN_POINT ( 'NONE',  ( 1.623707939105870413, -6.078451570951948213, 13.99999999999999645 ) ) ;
#885=CARTESIAN_POINT ( 'NONE',  ( -7.966005157978614193, 4.422220743486963812, 1.999999999999998224 ) ) ;
#887=CARTESIAN_POINT ( 'NONE',  ( -7.521311085815506559, -0.1255077825093695587, 1.999999999999998224 ) ) ;
#890=FILL_AREA_STYLE ('',( #2215 ) ) ;
#892=CARTESIAN_POINT ( 'NONE',  ( 1.730265954310492127, 6.073542049876722970, 1.999999999999998224 ) ) ;
#895=ORIENTED_EDGE ( 'NONE', *, *, #570, .T. ) ;
#898=CARTESIAN_POINT ( 'NONE',  ( 6.769338797470518365, 8.534199679355843671, 13.99999999999999645 ) ) ;
#903=CARTESIAN_POINT ( 'NONE',  ( -1.480145937554535385, 8.115026467927430431, 14.00000000000000000 ) ) ;
#904=CARTESIAN_POINT ( 'NONE',  ( -3.845892476879857025, 6.661954734853423155, 1.999999999999998224 ) ) ;
#906=CARTESIAN_POINT ( 'NONE',  ( 1.853537052132013807, -8.546502713975392851, 14.00000000000000000 ) ) ;
#908=CARTESIAN_POINT ( 'NONE',  ( 3.605080641954653053, -9.570177220923548944, 1.999999999999998224 ) ) ;
#909=CARTESIAN_POINT ( 'NONE',  ( -2.440069559021881496, 10.46881825416662259, 1.999999999999998224 ) ) ;
#911=CARTESIAN_POINT ( 'NONE',  ( -7.227555219266157849, -1.939125212622549999, 13.99999999999999645 ) ) ;
#913=CARTESIAN_POINT ( 'NONE',  ( -3.109042548464319378, -8.271822080922653697, 1.999999999999998224 ) ) ;
#914=CARTESIAN_POINT ( 'NONE',  ( -4.372214883940050534, 6.312905667202751481, 1.999999999999998224 ) ) ;
#919=CARTESIAN_POINT ( 'NONE',  ( 4.513069810084762601, -3.445129632735342451, 1.999999999999998224 ) ) ;
#930=CARTESIAN_POINT ( 'NONE',  ( -6.398096652174581678, -7.548242073784473760, 14.00000000000000000 ) ) ;
#931=CARTESIAN_POINT ( 'NONE',  ( -7.521311085815506559, -0.1255077825093695587, 1.999999999999998224 ) ) ;
#932=CARTESIAN_POINT ( 'NONE',  ( 5.059064342543293513, -7.053288479151686552, 1.999999999999998224 ) ) ;
#933=CARTESIAN_POINT ( 'NONE',  ( -7.892574838092353495, -1.309761382309196032, 14.00000000000000000 ) ) ;
#935=CARTESIAN_POINT ( 'NONE',  ( -3.798941939731882655, -9.621416145858376012, 1.999999999999998224 ) ) ;
#938=CARTESIAN_POINT ( 'NONE',  ( 3.426039378954557346, 5.938690629332270987, 13.99999999999999645 ) ) ;
#939=CARTESIAN_POINT ( 'NONE',  ( 1.147089839255700294, -8.682979827541576157, 1.999999999999998224 ) ) ;
#942=CARTESIAN_POINT ( 'NONE',  ( 3.892125705850321804, -6.036954802193386982, 1.999999999999998224 ) ) ;
#950=ORIENTED_EDGE ( 'NONE', *, *, #2485, .T. ) ;
#958=CARTESIAN_POINT ( 'NONE',  ( -10.03347820201837237, 0.3196629254998830660, 14.00000000000000000 ) ) ;
#959=CARTESIAN_POINT ( 'NONE',  ( -7.227555219266156072, -1.939125212622417660, 1.999999999999998224 ) ) ;
#961=CARTESIAN_POINT ( 'NONE',  ( -0.2798806129216870886, -8.779921314118375619, 1.999999999999998224 ) ) ;
#963=CARTESIAN_POINT ( 'NONE',  ( 7.379526280503350577, 5.862399640741291940, 14.00000000000000000 ) ) ;
#965=CARTESIAN_POINT ( 'NONE',  ( -8.741731599017841248, 6.051300285686449953, 1.999999999999998224 ) ) ;
#966=CARTESIAN_POINT ( 'NONE',  ( -1.336592501075063666, -5.709464570123372162, 14.00000000000000000 ) ) ;
#967=CARTESIAN_POINT ( 'NONE',  ( -7.763712483375483586, -3.368527140561099031, 13.99999999999999645 ) ) ;
#969=CARTESIAN_POINT ( 'NONE',  ( -7.521311085815508335, -0.1255077825093697530, 13.99999999999999645 ) ) ;
#970=CARTESIAN_POINT ( 'NONE',  ( -7.304208470130000741, 7.056621303511527721, 1.999999999999998224 ) ) ;
#973=CARTESIAN_POINT ( 'NONE',  ( 5.857810772706377733, -5.665644577056675679, 1.999999999999998224 ) ) ;
#979=CARTESIAN_POINT ( 'NONE',  ( -6.048456868091350636, 0.8014113234715940504, 1.999999999999998224 ) ) ;
#983=CARTESIAN_POINT ( 'NONE',  ( 7.456063200421762183, 7.959410280422752670, 13.99999999999999645 ) ) ;
#988=CARTESIAN_POINT ( 'NONE',  ( -5.391417556047953141, 8.653185861734563389, 14.00000000000000000 ) ) ;
#989=CARTESIAN_POINT ( 'NONE',  ( -6.762100275670003491, 3.470635719505328343, 1.999999999999998224 ) ) ;
#991=CARTESIAN_POINT ( 'NONE',  ( 3.810368753942602993, 7.433568398487427231, 1.999999999999998224 ) ) ;
#992=CARTESIAN_POINT ( 'NONE',  ( -9.031632682309723492, 0.1436733667526614300, 14.00000000000000000 ) ) ;
#994=CARTESIAN_POINT ( 'NONE',  ( -8.483256258862246213, -6.077987531410204980, 1.999999999999998224 ) ) ;
#996=CARTESIAN_POINT ( 'NONE',  ( -5.741039858921713979, -6.128965587877692300, 13.99999999999999645 ) ) ;
#997=CARTESIAN_POINT ( 'NONE',  ( -6.762100275670005267, 3.470635719505328787, 13.99999999999999645 ) ) ;
#999=CARTESIAN_POINT ( 'NONE',  ( -1.320393794063943860, 6.095439640211754551, 14.00000000000000000 ) ) ;
#1002=CARTESIAN_POINT ( 'NONE',  ( 9.020117466466054168, 0.2947087185667776055, 1.999999999999998224 ) ) ;
#1003=DIRECTION ( 'NONE',  ( 1.000000000000000000, 0.000000000000000000, 0.000000000000000000 ) ) ;
#1004=CARTESIAN_POINT ( 'NONE',  ( 6.340368144647110071, -1.697206311170896598, 1.999999999999998224 ) ) ;
#1006=CARTESIAN_POINT ( 'NONE',  ( 5.195030181282357162, -4.117271336869386289, 1.999999999999998224 ) ) ;
#1014=CARTESIAN_POINT ( 'NONE',  ( 9.123540010895988317, -2.926742269086383796, 14.00000000000000000 ) ) ;
#1015=CARTESIAN_POINT ( 'NONE',  ( 2.321214644803172078, -6.838859567843806886, 1.999999999999998224 ) ) ;
#1016=CARTESIAN_POINT ( 'NONE',  ( -8.290222237438479524, 3.747600907060152142, 1.999999999999998224 ) ) ;
#1017=CARTESIAN_POINT ( 'NONE',  ( 4.853468040355885194, -8.397360160973688537, 14.00000000000000000 ) ) ;
#1019=CARTESIAN_POINT ( 'NONE',  ( -10.53467355221071777, 0.3418899515810866485, 1.999999999999998224 ) ) ;
#1020=CARTESIAN_POINT ( 'NONE',  ( -1.320393794063943860, 6.095439640211754551, 14.00000000000000000 ) ) ;
#1021=CARTESIAN_POINT ( 'NONE',  ( -3.441860715206332522, -7.602597312514155270, 13.99999999999999645 ) ) ;
#1023=CARTESIAN_POINT ( 'NONE',  ( 8.269507991092025279, 6.356934974247397285, 1.999999999999998224 ) ) ;
#1025=CARTESIAN_POINT ( 'NONE',  ( -6.681468852107821377, -5.130140014479647625, 1.999999999999998224 ) ) ;
#1027=CARTESIAN_POINT ( 'NONE',  ( -6.734745854535898246, 2.161492950161982396, 1.999999999999998224 ) ) ;
#1029=CARTESIAN_POINT ( 'NONE',  ( -2.717942380035140104, -6.274577315194988181, 1.999999999999998224 ) ) ;
#1032=CARTESIAN_POINT ( 'NONE',  ( -6.762100275670003491, 3.470635719505328343, 1.999999999999998224 ) ) ;
#1038=CARTESIAN_POINT ( 'NONE',  ( -8.072272399573057200, -5.790267008922743486, 14.00000000000000000 ) ) ;
#1039=CARTESIAN_POINT ( 'NONE',  ( -7.884571930971327802, 3.418633173532902969, 1.999999999999998224 ) ) ;
#1041=CARTESIAN_POINT ( 'NONE',  ( -8.999716648909558359, -0.5976852874978595409, 1.999999999999998224 ) ) ;
#1042=CARTESIAN_POINT ( 'NONE',  ( 9.123540010895988317, -2.926742269086383796, 14.00000000000000000 ) ) ;
#1047=CARTESIAN_POINT ( 'NONE',  ( 2.389076732465380548, -5.237771676862081449, 14.00000000000000000 ) ) ;
#1048=CARTESIAN_POINT ( 'NONE',  ( -5.893815055328263774, 7.676334994785688259, 13.99999999999999645 ) ) ;
#1050=CARTESIAN_POINT ( 'NONE',  ( -5.183646570197097958, -3.010418922386785212, 14.00000000000000000 ) ) ;
#1052=CARTESIAN_POINT ( 'NONE',  ( -1.484422800923325125, -8.172499773499277254, 1.999999999999998224 ) ) ;
#1053=STYLED_ITEM('',(#5723),#2585);
#1057=CARTESIAN_POINT ( 'NONE',  ( -0.8347742375825081274, 7.207659102801795115, 1.999999999999998224 ) ) ;
#1060=CARTESIAN_POINT ( 'NONE',  ( -0.8347742375825081274, 7.207659102801795115, 1.999999999999998224 ) ) ;
#1071=CARTESIAN_POINT ( 'NONE',  ( 8.973806924230256499, -1.178693538871683488, 1.999999999999998224 ) ) ;
#1073=CARTESIAN_POINT ( 'NONE',  ( -3.672794075660469559, 8.451992513476518809, 1.999999999999998224 ) ) ;
#1074=CARTESIAN_POINT ( 'NONE',  ( 9.527640065891670673, 0.1642265212908743666, 14.00000000000000000 ) ) ;
#1079=CARTESIAN_POINT ( 'NONE',  ( -3.290073422422831406, -8.739709727799914063, 13.99999999999999645 ) ) ;
#1081=CARTESIAN_POINT ( 'NONE',  ( -7.559400777704422758, -6.425066744314571920, 1.999999999999998224 ) ) ;
#1084=CARTESIAN_POINT ( 'NONE',  ( 1.999247522871089311, 8.586038698136235325, 1.999999999999998224 ) ) ;
#1087=CARTESIAN_POINT ( 'NONE',  ( -3.595699629853521984, 5.016010494498948091, 1.999999999999998224 ) ) ;
#1089=CARTESIAN_POINT ( 'NONE',  ( 6.523553822664517554, -0.1051741892335503609, 1.999999999999998224 ) ) ;
#1095=B_SPLINE_CURVE_WITH_KNOTS ( 'NONE', 3,
 ( #1611, #3369, #2525, #1181, #307, #3854, #5523, #3340, #5580, #5606, #2876, #1208, #4709, #3421, #1691, #1233, #4739, #2558, #692, #2445, #256, #2015, #1581, #5092, #2906, #1725, #3052, #1749, #2672, #4024, #4399, #80, #5293, #51, #3532, #4424, #3940, #1836, #3081, #454, #3026, #2185, #4796, #5239, #942, #1352, #1296, #1805, #4826, #2583, #5665, #5321, #3110, #857, #4373, #428, #3593, #4859, #1381, #478, #3136, #887, #2267, #2213, #4342, #1032, #3564, #3505, #4884, #914, #5264, #2236, #2647, #1264, #4771, #3964, #2696, #24, #4451, #831, #393, #2154, #1776, #1320, #2613, #3991, #512, #3910, #3477, #1946, #1893, #4080, #4913, #973, #2731, #2378, #133, #4483, #2291, #3649, #221, #1052, #540, #1977, #5431, #5458, #2814, #1025, #1486, #4993, #564, #5405, #1434, #3699, #4538, #106, #3220, #2407, #2845, #3193, #3275, #2783, #1514, #4051, #4566, #4168, #5027, #1084, #4597, #3675, #628, #1862, #4943, #3618, #656, #594, #5346, #2759, #1002, #1403, #5377, #3165, #4512, #2320, #1463, #4967, #4113, #2347, #166, #1920, #3245, #4138, #193, #5144, #799, #1174, #2552, #2060, #2518, #301, #1204, #5118, #2468, #1635, #3731, #4313, #4652, #5517, #2010, #3417, #3820, #3762, #4282, #1603, #5055, #2436, #2093, #5575, #1576, #1140, #2899, #2035, #3363, #2494, #5168, #5545, #2927, #4733, #4679, #1113, #719, #335, #4226, #3850, #3393, #277, #4705, #740, #5490, #1551, #4250, #5602, #2954, #767, #1661, #4623, #363, #1229, #3790, #3333, #5084, #2986, #3305, #2870, #683, #4199, #249, #1686, #3443, #5200, #4853, #1260, #827, #46, #3987, #3020, #909, #3936, #2668, #2120, #3875, #1345, #2641, #4765, #2579, #5317, #4337, #4395, #1315, #450, #2690, #852 ),
 .UNSPECIFIED., .F., .F.,
 ( 4, 2, 2, 2, 2, 2, 2, 2, 2, 2, 2, 2, 2, 2, 2, 2, 2, 2, 2, 2, 2, 2, 2, 2, 2, 2, 2, 2, 2, 2, 2, 2, 2, 2, 2, 2, 2, 2, 2, 2, 2, 2, 2, 2, 2, 2, 2, 2, 2, 2, 2, 2, 2, 2, 2, 2, 2, 2, 2, 2, 2, 2, 2, 2, 2, 2, 2, 2, 2, 2, 2, 2, 2, 2, 2, 2, 2, 2, 2, 2, 2, 2, 2, 2, 2, 2, 2, 2, 2, 2, 2, 2, 2, 2, 2, 2, 2, 2, 2, 2, 2, 2, 2, 2, 2, 2, 2, 2, 2, 2, 2, 2, 2, 2, 2, 2, 2, 2, 2, 2, 4 ),
 ( 0.000000000000000000, 0.01562500000000000000, 0.03125000000000000000, 0.04687500000000000000, 0.06250000000000000000, 0.07812500000000000000, 0.09375000000000000000, 0.1093750000000000000, 0.1250000000000000000, 0.1328125000000000000, 0.1406250000000000000, 0.1484375000000000000, 0.1562500000000000000, 0.1640625000000000000, 0.1718750000000000000, 0.1796875000000000000, 0.1875000000000000000, 0.1953125000000000000, 0.2031250000000000000, 0.2109375000000000000, 0.2187500000000000000, 0.2265625000000000000, 0.2343750000000000000, 0.2421875000000000000, 0.2500000000000000000, 0.2578125000000000000, 0.2656250000000000000, 0.2734375000000000000, 0.2812500000000000000, 0.2890625000000000000, 0.2968750000000000000, 0.3046875000000000000, 0.3125000000000000000, 0.3203125000000000000, 0.3281250000000000000, 0.3359375000000000000, 0.3437500000000000000, 0.3515625000000000000, 0.3593750000000000000, 0.3671875000000000000, 0.3750000000000000000, 0.3828125000000000000, 0.3906250000000000000, 0.3984375000000000000, 0.4062500000000000000, 0.4140625000000000000, 0.4218750000000000000, 0.4296875000000000000, 0.4375000000000000000, 0.4453125000000000000, 0.4531250000000000000, 0.4609375000000000000, 0.4687500000000000000, 0.4765625000000000000, 0.4843750000000000000, 0.4921875000000000000, 0.5000000000000000000, 0.5078125000000000000, 0.5156250000000000000, 0.5234375000000000000, 0.5312500000000000000, 0.5390625000000000000, 0.5468750000000000000, 0.5546875000000000000, 0.5625000000000000000, 0.5703125000000000000, 0.5781250000000000000, 0.5859375000000000000, 0.5937500000000000000, 0.6015625000000000000, 0.6093750000000000000, 0.6171875000000000000, 0.6250000000000000000, 0.6328125000000000000, 0.6406250000000000000, 0.6484375000000000000, 0.6562500000000000000, 0.6640625000000000000, 0.6718750000000000000, 0.6796875000000000000, 0.6875000000000000000, 0.6953125000000000000, 0.7031250000000000000, 0.7109375000000000000, 0.7187500000000000000, 0.7265625000000000000, 0.7343750000000000000, 0.7421875000000000000, 0.7500000000000000000, 0.7578125000000000000, 0.7656250000000000000, 0.7734375000000000000, 0.7812500000000000000, 0.7890625000000000000, 0.7968750000000000000, 0.8046875000000000000, 0.8125000000000000000, 0.8203125000000000000, 0.8281250000000000000, 0.8359375000000000000, 0.8437500000000000000, 0.8515625000000000000, 0.8593750000000000000, 0.8671875000000000000, 0.8750000000000000000, 0.8828125000000000000, 0.8906250000000000000, 0.8984375000000000000, 0.9062500000000000000, 0.9140625000000000000, 0.9218750000000000000, 0.9296875000000000000, 0.9375000000000000000, 0.9453125000000000000, 0.9531250000000000000, 0.9609375000000000000, 0.9687500000000000000, 0.9765625000000000000, 0.9843750000000000000, 0.9921875000000000000, 1.000000000000000000 ),
 .UNSPECIFIED. ) ;
#1099=CARTESIAN_POINT ( 'NONE',  ( 10.50003631213658117, 0.006025845833179007717, 14.00000000000000000 ) ) ;
#1100=CARTESIAN_POINT ( 'NONE',  ( 1.954797901281672967, -9.037865403626939909, 1.999999999999998224 ) ) ;
#1102=CARTESIAN_POINT ( 'NONE',  ( -7.884571930971329579, 3.418633173532294123, 13.99999999999999645 ) ) ;
#1105=LINE ( 'NONE', #4672, #511 ) ;
#1108=CARTESIAN_POINT ( 'NONE',  ( 5.648567055624232225, 4.800053419556652656, 14.00000000000000000 ) ) ;
#1109=CARTESIAN_POINT ( 'NONE',  ( -2.557952627993306471, -8.967547948949398773, 13.99999999999999645 ) ) ;
#1111=CARTESIAN_POINT ( 'NONE',  ( 5.460516619045268527, 3.400499599735717915, 14.00000000000000000 ) ) ;
#1113=CARTESIAN_POINT ( 'NONE',  ( 10.02932042447482175, 0.1670047327945775040, 1.999999999999998224 ) ) ;
#1116=CARTESIAN_POINT ( 'NONE',  ( 1.730265954310492127, 6.073542049876722970, 1.999999999999998224 ) ) ;
#1118=CARTESIAN_POINT ( 'NONE',  ( -6.881333183080980298, -1.254343363641173381, 1.999999999999998224 ) ) ;
#1120=CARTESIAN_POINT ( 'NONE',  ( -1.451466707715608040, -6.203196315423898710, 13.99999999999999645 ) ) ;
#1124=EDGE_LOOP ( 'NONE', ( #4217, #5409, #2571, #1945 ) ) ;
#1127=CARTESIAN_POINT ( 'NONE',  ( -8.388197440586290909, -1.387539741535495974, 1.999999999999998224 ) ) ;
#1128=CARTESIAN_POINT ( 'NONE',  ( -1.565980662507674648, 8.609317438862776228, 13.99999999999999645 ) ) ;
#1129=CARTESIAN_POINT ( 'NONE',  ( 1.837295235934470528, 10.14794156482770404, 14.00000000000000000 ) ) ;
#1134=CARTESIAN_POINT ( 'NONE',  ( 6.268835244667308793, -4.335177162149436825, 14.00000000000000000 ) ) ;
#1135=CARTESIAN_POINT ( 'NONE',  ( -9.406456921418632433, 1.708717176649267477, 13.99999999999999645 ) ) ;
#1137=CARTESIAN_POINT ( 'NONE',  ( 0.9466184546083361573, 7.233353930637703044, 14.00000000000000000 ) ) ;
#1140=CARTESIAN_POINT ( 'NONE',  ( 3.158576809044846279, 9.313732666428188978, 1.999999999999998224 ) ) ;
#1145=CARTESIAN_POINT ( 'NONE',  ( -6.281085993838467552, -4.827840781182768382, 1.999999999999998224 ) ) ;
#1147=CARTESIAN_POINT ( 'NONE',  ( -3.813875884798381577, -6.869235835554530212, 1.999999999999998224 ) ) ;
#1151=CARTESIAN_POINT ( 'NONE',  ( -2.122668041763332347, 7.434468402752584026, 13.99999999999999645 ) ) ;
#1153=LINE ( 'NONE', #4124, #1162 ) ;
#1159=CARTESIAN_POINT ( 'NONE',  ( -6.681468852107821377, -5.130140014479647625, 1.999999999999998224 ) ) ;
#1161=CARTESIAN_POINT ( 'NONE',  ( 6.401046915552173644, 6.194151307163302533, 13.99999999999999645 ) ) ;
#1162=VECTOR ( 'NONE', #666, 1000.000000000000000 ) ;
#1168=CARTESIAN_POINT ( 'NONE',  ( 6.592258996018688144, -3.799026305082323418, 14.00000000000000000 ) ) ;
#1169=CARTESIAN_POINT ( 'NONE',  ( 10.02239396097876423, -0.6576683464575836524, 13.99999999999999645 ) ) ;
#1171=CARTESIAN_POINT ( 'NONE',  ( 6.680730669075651385, 3.301097878975988831, 14.00000000000000000 ) ) ;
#1174=CARTESIAN_POINT ( 'NONE',  ( -4.679820741051314847, -8.111215689328634681, 1.999999999999998224 ) ) ;
#1180=CARTESIAN_POINT ( 'NONE',  ( 7.526353627798827439, -0.2404185136226760222, 1.999999999999998224 ) ) ;
#1181=CARTESIAN_POINT ( 'NONE',  ( 4.914575889516862972, -3.754581871930560144, 1.999999999999998224 ) ) ;
#1182=CARTESIAN_POINT ( 'NONE',  ( 6.804422688527093754, 1.586354726854036112, 13.99999999999999645 ) ) ;
#1184=CARTESIAN_POINT ( 'NONE',  ( 7.258279873955303607, -6.354128476750924293, 1.999999999999998224 ) ) ;
#1190=CARTESIAN_POINT ( 'NONE',  ( -9.026614039607443019, -2.903226997913650465, 1.999999999999998224 ) ) ;
#1192=CARTESIAN_POINT ( 'NONE',  ( 9.650319724629330409, 2.588775111615905011, 13.99999999999999645 ) ) ;
#1193=CARTESIAN_POINT ( 'NONE',  ( 10.36702220812670028, 1.720931399333114120, 14.00000000000000000 ) ) ;
#1199=CARTESIAN_POINT ( 'NONE',  ( -6.065725208710916583, -3.376743199310593635, 14.00000000000000000 ) ) ;
#1200=CARTESIAN_POINT ( 'NONE',  ( 5.279590631142085044, 9.498297537455629325, 13.99999999999999645 ) ) ;
#1201=CARTESIAN_POINT ( 'NONE',  ( 7.526353627798829216, -0.2404185136226759112, 14.00000000000000000 ) ) ;
#1204=CARTESIAN_POINT ( 'NONE',  ( -8.411612136543093143, -4.319922787977411360, 1.999999999999998224 ) ) ;
#1207=CARTESIAN_POINT ( 'NONE',  ( 7.439669587982602472, 0.9822684312230360870, 1.999999999999998224 ) ) ;
#1208=CARTESIAN_POINT ( 'NONE',  ( -5.623512120026769701, -3.262381593762911258, 1.999999999999998224 ) ) ;
#1209=CARTESIAN_POINT ( 'NONE',  ( 1.649120185255091187, 7.633850905136058351, 13.99999999999999645 ) ) ;
#1212=CARTESIAN_POINT ( 'NONE',  ( -1.515482495401827556, 9.129776367296644324, 1.999999999999998224 ) ) ;
#1218=CARTESIAN_POINT ( 'NONE',  ( -1.592064345877354903, 9.625584969239746158, 13.99999999999999645 ) ) ;
#1219=CARTESIAN_POINT ( 'NONE',  ( 6.452733273991772656, 8.145031704320798482, 14.00000000000000000 ) ) ;
#1225=CARTESIAN_POINT ( 'NONE',  ( 7.526353627798829216, -0.2404185136226759112, 14.00000000000000000 ) ) ;
#1226=CARTESIAN_POINT ( 'NONE',  ( 0.1774200004017887078, 10.78715707688374614, 13.99999999999999645 ) ) ;
#1227=CARTESIAN_POINT ( 'NONE',  ( -6.317162512442926037, 3.238855812894408714, 14.00000000000000000 ) ) ;
#1229=CARTESIAN_POINT ( 'NONE',  ( -6.045729098460860484, -8.441868823237593134, 1.999999999999998224 ) ) ;
#1232=CARTESIAN_POINT ( 'NONE',  ( -2.138212235155099616, 7.953261502403489835, 1.999999999999998224 ) ) ;
#1233=CARTESIAN_POINT ( 'NONE',  ( -5.978927507574433697, 2.933119789328457294, 1.999999999999998224 ) ) ;
#1234=CARTESIAN_POINT ( 'NONE',  ( 3.892125705850195683, -6.036954802193643665, 13.99999999999999645 ) ) ;
#1236=CARTESIAN_POINT ( 'NONE',  ( -5.748891254250207083, -8.037420881456807109, 1.999999999999998224 ) ) ;
#1244=CARTESIAN_POINT ( 'NONE',  ( 3.388254439433305176, -8.575817650944683734, 13.99999999999999645 ) ) ;
#1253=CARTESIAN_POINT ( 'NONE',  ( -2.020383375745357313, -7.552201994671271734, 14.00000000000000000 ) ) ;
#1254=CARTESIAN_POINT ( 'NONE',  ( 10.86297249782086105, 1.796588950249321304, 13.99999999999999645 ) ) ;
#1257=CARTESIAN_POINT ( 'NONE',  ( 4.415008247871436531, 7.106745273741267965, 14.00000000000000000 ) ) ;
#1260=CARTESIAN_POINT ( 'NONE',  ( -7.660583958272733973, 7.409732212660907535, 1.999999999999998224 ) ) ;
#1261=CARTESIAN_POINT ( 'NONE',  ( 6.209839678909983895, -3.451293940533043614, 13.99999999999999645 ) ) ;
#1263=CARTESIAN_POINT ( 'NONE',  ( -7.892574838092051515, -1.309761382309195366, 1.999999999999998224 ) ) ;
#1264=CARTESIAN_POINT ( 'NONE',  ( -0.8890388043606449742, 7.706404363472288743, 1.999999999999998224 ) ) ;
#1266=CARTESIAN_POINT ( 'NONE',  ( -3.989331152809451275, -6.191695749071043586, 13.99999999999999645 ) ) ;
#1269=CARTESIAN_POINT ( 'NONE',  ( 6.863489721961431478, 6.439594285167053123, 1.999999999999998224 ) ) ;
#1279=CARTESIAN_POINT ( 'NONE',  ( 9.843274586260610803, 1.790275038161259991, 13.99999999999999645 ) ) ;
#1285=CARTESIAN_POINT ( 'NONE',  ( 5.059064342543619475, -7.053288479152013402, 14.00000000000000000 ) ) ;
#1287=CARTESIAN_POINT ( 'NONE',  ( -7.660583958272733973, 7.409732212661285011, 13.99999999999999645 ) ) ;
#1289=CARTESIAN_POINT ( 'NONE',  ( 8.453438707197836521, 0.9797652757261499090, 14.00000000000000000 ) ) ;
#1292=CARTESIAN_POINT ( 'NONE',  ( -0.4015567206216588692, -6.330257989742014146, 13.99999999999999645 ) ) ;
#1294=CARTESIAN_POINT ( 'NONE',  ( 0.7514524083000287957, 9.263466152294371980, 1.999999999999998224 ) ) ;
#1296=CARTESIAN_POINT ( 'NONE',  ( 2.321214644803172078, -6.838859567843806886, 1.999999999999998224 ) ) ;
#1297=CARTESIAN_POINT ( 'NONE',  ( -3.594774944545354955, 7.935102286574237773, 13.99999999999999645 ) ) ;
#1304=CARTESIAN_POINT ( 'NONE',  ( -7.035243215357270152, 8.023489478516461659, 13.99999999999999645 ) ) ;
#1309=CARTESIAN_POINT ( 'NONE',  ( -1.390902631672706224, -7.679604985168660747, 14.00000000000000000 ) ) ;
#1310=CARTESIAN_POINT ( 'NONE',  ( 6.000000000000000000, 0.000000000000000000, 1.999999999999998224 ) ) ;
#1313=CARTESIAN_POINT ( 'NONE',  ( 1.881113203117336319, 8.098457488330069509, 14.00000000000000000 ) ) ;
#1315=CARTESIAN_POINT ( 'NONE',  ( 10.40193138080405255, 3.529992181067783452, 1.999999999999998224 ) ) ;
#1316=CARTESIAN_POINT ( 'NONE',  ( -5.432680616552289621, 3.899654942172362748, 14.00000000000093792 ) ) ;
#1318=CARTESIAN_POINT ( 'NONE',  ( 5.710084532570392390, 7.448680193042510389, 1.999999999999998224 ) ) ;
#1320=CARTESIAN_POINT ( 'NONE',  ( 7.132151089625187623, 3.519983721611797733, 1.999999999999998224 ) ) ;
#1323=CARTESIAN_POINT ( 'NONE',  ( 6.452733273992156349, 8.145031704320794930, 1.999999999999998224 ) ) ;
#1324=CARTESIAN_POINT ( 'NONE',  ( -5.637968025906138436, -2.116521738900817073, 1.999999999999998224 ) ) ;
#1329=CARTESIAN_POINT ( 'NONE',  ( -9.197478219253614640, 5.306711421960436326, 13.99999999999999645 ) ) ;
#1336=AXIS2_PLACEMENT_3D ( 'NONE', #283, #2997, #5213 ) ;
#1337=CARTESIAN_POINT ( 'NONE',  ( -6.281085993838468440, -4.827840781183066809, 14.00000000000000000 ) ) ;
#1338=CARTESIAN_POINT ( 'NONE',  ( -7.211577653563208123, 2.317451195016654530, 1.999999999999998224 ) ) ;
#1341=CARTESIAN_POINT ( 'NONE',  ( -3.987536574861253236, 7.161134007378101352, 14.00000000000000000 ) ) ;
#1344=CARTESIAN_POINT ( 'NONE',  ( 5.099673838352487998, -8.834479793761566668, 1.999999999999998224 ) ) ;
#1345=CARTESIAN_POINT ( 'NONE',  ( 4.476660083460862971, 9.887553134099890784, 1.999999999999998224 ) ) ;
#1347=CARTESIAN_POINT ( 'NONE',  ( -3.989331152809451275, -6.191695749071043586, 13.99999999999999645 ) ) ;
#1349=CARTESIAN_POINT ( 'NONE',  ( 8.618507686538960044, 3.909830026711944573, 1.999999999999998224 ) ) ;
#1352=CARTESIAN_POINT ( 'NONE',  ( 2.869471237997587743, -6.613103333303327780, 1.999999999999998224 ) ) ;
#1356=CARTESIAN_POINT ( 'NONE',  ( 5.326024957120312209, -1.813589758486610970, 1.999999999999998224 ) ) ;
#1358=CARTESIAN_POINT ( 'NONE',  ( 5.733165789232423037, 2.946509839760266924, 1.999999999999998224 ) ) ;
#1364=CARTESIAN_POINT ( 'NONE',  ( -9.742306995815035009, -3.848972158781221786, 13.99999999999999645 ) ) ;
#1370=CARTESIAN_POINT ( 'NONE',  ( 8.618507686539667034, 3.909830026712121764, 14.00000000000000000 ) ) ;
#1371=CARTESIAN_POINT ( 'NONE',  ( 2.869471237997587743, -6.613103333303327780, 1.999999999999998224 ) ) ;
#1372=CARTESIAN_POINT ( 'NONE',  ( 6.929006764466009827, 4.804313515625705300, 1.999999999999998224 ) ) ;
#1373=CARTESIAN_POINT ( 'NONE',  ( -7.425829140954380847, 3.215541426300493111, 14.00000000000000000 ) ) ;
#1375=CARTESIAN_POINT ( 'NONE',  ( 0.3355163285737912116, -10.27362971114624024, 1.999999999999998224 ) ) ;
#1377=CARTESIAN_POINT ( 'NONE',  ( 6.000000000000001776, 0.000000000000000000, 13.99999999999999645 ) ) ;
#1379=CARTESIAN_POINT ( 'NONE',  ( 0.3244988297792679166, -9.772062696132405080, 1.999999999999998224 ) ) ;
#1381=CARTESIAN_POINT ( 'NONE',  ( -6.792624376349762905, -3.077375260546124203, 1.999999999999998224 ) ) ;
#1384=CARTESIAN_POINT ( 'NONE',  ( 9.925004466820084303, 3.374327561486830884, 1.999999999999998224 ) ) ;
#1389=CARTESIAN_POINT ( 'NONE',  ( 9.599547022228486881, -3.085197981543154278, 13.99999999999999645 ) ) ;
#1393=CARTESIAN_POINT ( 'NONE',  ( -4.354965481614498479, -8.841480220785717492, 14.00000000000000000 ) ) ;
#1394=CARTESIAN_POINT ( 'NONE',  ( -5.322107489685658166, 5.499660323246576610, 1.999999999999998224 ) ) ;
#1395=CARTESIAN_POINT ( 'NONE',  ( 3.857245400775495714, -7.804869966781508239, 1.999999999999998224 ) ) ;
#1396=CARTESIAN_POINT ( 'NONE',  ( 2.992331685656917539, 8.840389773664524498, 14.00000000000000000 ) ) ;
#1398=CARTESIAN_POINT ( 'NONE',  ( 10.02932042447482175, 0.1670047327945775040, 1.999999999999998224 ) ) ;
#1400=CARTESIAN_POINT ( 'NONE',  ( 7.992346231215207375, -0.9198489573344114101, 13.99999999999999645 ) ) ;
#1401=CARTESIAN_POINT ( 'NONE',  ( -5.322107489685387272, 5.499660323246577498, 13.99999999999999645 ) ) ;
#1402=CARTESIAN_POINT ( 'NONE',  ( 3.713512749562912774, 8.576920285552665391, 1.999999999999998224 ) ) ;
#1403=CARTESIAN_POINT ( 'NONE',  ( 8.973806924230256499, -1.178693538871683488, 1.999999999999998224 ) ) ;
#1409=CARTESIAN_POINT ( 'NONE',  ( 0.2014543481397604585, 6.272771216426899166, 1.999999999999998224 ) ) ;
#1412=CARTESIAN_POINT ( 'NONE',  ( -3.287100391418014578, 10.22059872437975869, 13.99999999999999645 ) ) ;
#1417=ORIENTED_EDGE ( 'NONE', *, *, #570, .F. ) ;
#1418=CARTESIAN_POINT ( 'NONE',  ( 8.172274133038307298, -5.076547540501183065, 14.00000000000000000 ) ) ;
#1419=CARTESIAN_POINT ( 'NONE',  ( 5.194219494279652238, 4.554949839096303243, 1.999999999999998224 ) ) ;
#1422=CARTESIAN_POINT ( 'NONE',  ( -2.415560149437878668, -8.486491385245608754, 1.999999999999998224 ) ) ;
#1424=CARTESIAN_POINT ( 'NONE',  ( -7.161907081466633684, 5.673982509929174967, 14.00000000000000000 ) ) ;
#1426=CARTESIAN_POINT ( 'NONE',  ( -1.342170334697201595, -10.21728332006300199, 1.999999999999998224 ) ) ;
#1428=CARTESIAN_POINT ( 'NONE',  ( 8.952336951391263398, 1.032601321559317276, 13.99999999999999645 ) ) ;
#1430=CARTESIAN_POINT ( 'NONE',  ( -0.2539011084976132149, 7.766605221862832309, 13.99999999999999645 ) ) ;
#1431=CARTESIAN_POINT ( 'NONE',  ( -2.744490807750914918, 5.556819979548927257, 14.00000000000000000 ) ) ;
#1434=CARTESIAN_POINT ( 'NONE',  ( -8.486979168634645632, -0.6954046021538184963, 1.999999999999998224 ) ) ;
#1439=CARTESIAN_POINT ( 'NONE',  ( 6.004028658818956643, -2.715480180205985583, 1.999999999999998224 ) ) ;
#1444=CARTESIAN_POINT ( 'NONE',  ( -6.112420884766619267, -2.295018720694776970, 13.99999999999999645 ) ) ;
#1451=CARTESIAN_POINT ( 'NONE',  ( 9.164356920906893578, 2.464151434935829332, 14.00000000000000000 ) ) ;
#1452=CARTESIAN_POINT ( 'NONE',  ( 5.213743241621227931, -4.883528188333804643, 1.999999999999998224 ) ) ;
#1455=CARTESIAN_POINT ( 'NONE',  ( -6.826495404309643966, 4.393449859560456083, 1.999999999999998224 ) ) ;
#1456=CARTESIAN_POINT ( 'NONE',  ( 1.511842404626676961, 9.183516746439467582, 14.00000000000000000 ) ) ;
#1458=CARTESIAN_POINT ( 'NONE',  ( 7.066195124645999748, -7.302433507960749637, 1.999999999999998224 ) ) ;
#1459=CARTESIAN_POINT ( 'NONE',  ( -6.069783318623454882, -0.2142533344233820691, 14.00000000000000000 ) ) ;
#1460=CARTESIAN_POINT ( 'NONE',  ( 8.027649061864064350, -0.2602747315786822502, 13.99999999999999645 ) ) ;
#1461=CARTESIAN_POINT ( 'NONE',  ( 7.108868828250527905, 7.597268273414325535, 1.999999999999998224 ) ) ;
#1463=CARTESIAN_POINT ( 'NONE',  ( 6.971023843911450690, -5.915260676233723203, 1.999999999999998224 ) ) ;
#1466=CARTESIAN_POINT ( 'NONE',  ( 5.460516619045266751, 3.400499599735594014, 1.999999999999998224 ) ) ;
#1469=CARTESIAN_POINT ( 'NONE',  ( -6.742266116715657454, -1.811900715329134215, 1.999999999999998224 ) ) ;
#1471=CARTESIAN_POINT ( 'NONE',  ( 4.914575889516433094, -3.754581871930561032, 13.99999999999999645 ) ) ;
#1475=CARTESIAN_POINT ( 'NONE',  ( 9.348788865899230416, 1.705571004836294646, 14.00000000000000000 ) ) ;
#1476=CARTESIAN_POINT ( 'NONE',  ( -2.153669193480073574, -8.035861145135083206, 1.999999999999998224 ) ) ;
#1477=CARTESIAN_POINT ( 'NONE',  ( 7.017208779832875720, -5.019401656906101294, 1.999999999999998224 ) ) ;
#1478=CARTESIAN_POINT ( 'NONE',  ( -2.970508497641844325, 8.737606122599315128, 14.00000000000000000 ) ) ;
#1482=CARTESIAN_POINT ( 'NONE',  ( 3.622712361020366867, 5.236663886535375845, 14.00000000000000000 ) ) ;
#1483=CARTESIAN_POINT ( 'NONE',  ( -1.484422800923361985, -8.172499773498691056, 13.99999999999999645 ) ) ;
#1484=CARTESIAN_POINT ( 'NONE',  ( 8.774740126074938473, 5.663528079765400847, 1.999999999999998224 ) ) ;
#1486=CARTESIAN_POINT ( 'NONE',  ( -7.091148812992122963, -4.571561645352110403, 1.999999999999998224 ) ) ;
#1488=CARTESIAN_POINT ( 'NONE',  ( 4.062840028443489793, -5.287223670286648414, 1.999999999999998224 ) ) ;
#1490=CARTESIAN_POINT ( 'NONE',  ( -7.019651866617071079, -0.1200674265790944856, 1.999999999999998224 ) ) ;
#1492=CARTESIAN_POINT ( 'NONE',  ( 5.806279480218260680, -1.975834710110475401, 13.99999999999999645 ) ) ;
#1499=CARTESIAN_POINT ( 'NONE',  ( 7.748217264256983761, 4.472783157626249562, 1.999999999999998224 ) ) ;
#1501=CARTESIAN_POINT ( 'NONE',  ( 0.7514524083000287957, 9.263466152294371980, 1.999999999999998224 ) ) ;
#1502=CARTESIAN_POINT ( 'NONE',  ( 5.071900148311402567, 7.881338450277072027, 14.00000000000000000 ) ) ;
#1505=CARTESIAN_POINT ( 'NONE',  ( 6.769338797470902946, 8.534199679356609280, 1.999999999999998224 ) ) ;
#1508=CARTESIAN_POINT ( 'NONE',  ( 6.019515613300196577, 7.843576796802396167, 13.99999999999999645 ) ) ;
#1511=CARTESIAN_POINT ( 'NONE',  ( -3.922355934210178585, -4.464780306277046584, 14.00000000000000000 ) ) ;
#1514=CARTESIAN_POINT ( 'NONE',  ( -3.594774944545354511, 7.935102286573618713, 1.999999999999998224 ) ) ;
#1519=CARTESIAN_POINT ( 'NONE',  ( -5.525185448606692695, 2.707100724334796649, 1.999999999999998224 ) ) ;
#1522=CARTESIAN_POINT ( 'NONE',  ( 7.280083392764698402, -2.072676875633882254, 1.999999999999998224 ) ) ;
#1534=CARTESIAN_POINT ( 'NONE',  ( -6.848710654519973851, 5.255840572796829591, 1.999999999999998224 ) ) ;
#1537=CARTESIAN_POINT ( 'NONE',  ( 0.5432484998931954578, -8.249156888542636068, 13.99999999999999645 ) ) ;
#1538=CARTESIAN_POINT ( 'NONE',  ( 9.320190601379009010, -2.164585516638707574, 1.999999999999998224 ) ) ;
#1546=CARTESIAN_POINT ( 'NONE',  ( 4.776808680784973227, 5.634249062854204126, 14.00000000000000000 ) ) ;
#1547=CARTESIAN_POINT ( 'NONE',  ( 7.422282976138728117, -5.315384720684047437, 13.99999999999999645 ) ) ;
#1549=CARTESIAN_POINT ( 'NONE',  ( 2.672042568001582907, -6.151894458592797932, 14.00000000000000000 ) ) ;
#1551=CARTESIAN_POINT ( 'NONE',  ( 3.605080641954653053, -9.570177220923548944, 1.999999999999998224 ) ) ;
#1555=CARTESIAN_POINT ( 'NONE',  ( 0.5542950790998156796, -6.736796398737814329, 1.999999999999998224 ) ) ;
#1557=CARTESIAN_POINT ( 'NONE',  ( 1.760389272475360256, -7.536528230137968798, 1.999999999999998224 ) ) ;
#1565=CARTESIAN_POINT ( 'NONE',  ( 4.074896204546095468, -8.256886768008961042, 1.999999999999998224 ) ) ;
#1566=CARTESIAN_POINT ( 'NONE',  ( -4.227552200850896114, 7.601683304540504338, 13.99999999999999645 ) ) ;
#1572=CARTESIAN_POINT ( 'NONE',  ( -5.370374743919055227, 4.702532619530572333, 14.00000000000000000 ) ) ;
#1573=CARTESIAN_POINT ( 'NONE',  ( 7.775655769254120386, 6.170250810330326630, 13.99999999999999645 ) ) ;
#1574=CARTESIAN_POINT ( 'NONE',  ( -5.370374743919055227, 4.702532619530572333, 14.00000000000000000 ) ) ;
#1576=CARTESIAN_POINT ( 'NONE',  ( 1.598519525623709248, 9.677660462521251006, 1.999999999999998224 ) ) ;
#1578=CARTESIAN_POINT ( 'NONE',  ( 3.520917041835318173, -6.848083076130971669, 1.999999999999998224 ) ) ;
#1580=CARTESIAN_POINT ( 'NONE',  ( -1.390902631672706002, -7.679604985168658970, 1.999999999999998224 ) ) ;
#1581=CARTESIAN_POINT ( 'NONE',  ( -0.8811140424828312057, 6.693995663234410642, 1.999999999999998224 ) ) ;
#1582=CARTESIAN_POINT ( 'NONE',  ( -3.886954398759500773, 5.424498719065526053, 13.99999999999999645 ) ) ;
#1583=STYLED_ITEM ( 'NONE', ( #4887 ), #1852 ) ;
#1589=CARTESIAN_POINT ( 'NONE',  ( -8.513020831365363250, 0.6954046021538080602, 1.999999999999998224 ) ) ;
#1590=CARTESIAN_POINT ( 'NONE',  ( -7.211577653563209900, 2.317451195016654975, 13.99999999999999645 ) ) ;
#1591=CARTESIAN_POINT ( 'NONE',  ( 2.667884741302309681, 9.975564253400266423, 14.00000000000000000 ) ) ;
#1596=CARTESIAN_POINT ( 'NONE',  ( 7.439669587982604249, 0.9822684312230363091, 14.00000000000000000 ) ) ;
#1598=CARTESIAN_POINT ( 'NONE',  ( -8.017392084630589721, -4.988806607527435766, 13.99999999999999645 ) ) ;
#1600=CARTESIAN_POINT ( 'NONE',  ( 6.034497645749724803, 4.327592090611794617, 14.00000000000000000 ) ) ;
#1603=CARTESIAN_POINT ( 'NONE',  ( -3.867583043141952892, 8.914321633328466277, 1.999999999999998224 ) ) ;
#1607=CARTESIAN_POINT ( 'NONE',  ( 1.881113203117336097, 8.098457488329447784, 1.999999999999998224 ) ) ;
#1611=CARTESIAN_POINT ( 'NONE',  ( 6.000000000000000000, 0.000000000000000000, 1.999999999999998224 ) ) ;
#1612=CARTESIAN_POINT ( 'NONE',  ( -2.965071238690786259, 6.007415411094351398, 13.99999999999999645 ) ) ;
#1619=CARTESIAN_POINT ( 'NONE',  ( 8.774740126074163982, 5.663528079765788981, 14.00000000000000000 ) ) ;
#1620=CARTESIAN_POINT ( 'NONE',  ( -6.537688394901212341, -6.759197365500154930, 1.999999999999998224 ) ) ;
#1621=CARTESIAN_POINT ( 'NONE',  ( 3.917689075872249571, 9.035181080458080771, 13.99999999999999645 ) ) ;
#1624=CARTESIAN_POINT ( 'NONE',  ( 10.48651993945768623, 0.8648464362367445091, 14.00000000000000000 ) ) ;
#1629=CARTESIAN_POINT ( 'NONE',  ( 2.672042568001582907, -6.151894458592797932, 14.00000000000000000 ) ) ;
#1630=CARTESIAN_POINT ( 'NONE',  ( -5.432680616545222385, 3.899654942179428652, 2.000000000001176392 ) ) ;
#1632=CARTESIAN_POINT ( 'NONE',  ( -3.715337444063475658, -5.771435016728993617, 14.00000000000000000 ) ) ;
#1635=CARTESIAN_POINT ( 'NONE',  ( -9.500632974892678106, -0.6255030753161154866, 1.999999999999998224 ) ) ;
#1640=CARTESIAN_POINT ( 'NONE',  ( 5.648567055624510225, 4.800053419556092216, 1.999999999999998224 ) ) ;
#1642=CARTESIAN_POINT ( 'NONE',  ( -5.745624475482375537, 5.035517847229356470, 13.99999999999999645 ) ) ;
#1644=CARTESIAN_POINT ( 'NONE',  ( -5.592500163775054212, 7.275211197852026856, 1.999999999999998224 ) ) ;
#1650=CARTESIAN_POINT ( 'NONE',  ( -5.250997584835957355, 8.145342823909338392, 13.99999999999999645 ) ) ;
#1652=CARTESIAN_POINT ( 'NONE',  ( 9.602236826902712963, 4.172718697305597857, 14.00000000000000000 ) ) ;
#1657=CARTESIAN_POINT ( 'NONE',  ( 5.195030181282107584, -4.117271336869512410, 14.00000000000000000 ) ) ;
#1658=CARTESIAN_POINT ( 'NONE',  ( -6.551010013419180211, 0.8677952034721564400, 1.999999999999998224 ) ) ;
#1659=CARTESIAN_POINT ( 'NONE',  ( 1.540339863274486465, 7.144097608501355445, 14.00000000000000000 ) ) ;
#1661=CARTESIAN_POINT ( 'NONE',  ( -2.179108132477198367, -10.08557389312680108, 1.999999999999998224 ) ) ;
#1664=CARTESIAN_POINT ( 'NONE',  ( 7.925371078819430259, 2.990572132494937474, 1.999999999999998224 ) ) ;
#1666=CARTESIAN_POINT ( 'NONE',  ( 3.471913601335457233, 7.039518430846527508, 13.99999999999999645 ) ) ;
#1669=CARTESIAN_POINT ( 'NONE',  ( -4.668631340267960894, 9.078485505801564770, 1.999999999999998224 ) ) ;
#1675=CARTESIAN_POINT ( 'NONE',  ( -9.500632974893353122, -0.6255030753161997525, 13.99999999999999645 ) ) ;
#1678=DIRECTION ( 'NONE',  ( 2.891205793294678326E-16, -1.129377263005733721E-18, 1.000000000000000000 ) ) ;
#1681=CARTESIAN_POINT ( 'NONE',  ( 0.5141566911144540564, -7.748312628312728378, 14.00000000000000000 ) ) ;
#1682=CARTESIAN_POINT ( 'NONE',  ( 4.476660083460862971, 9.887553134100658170, 13.99999999999999645 ) ) ;
#1684=CARTESIAN_POINT ( 'NONE',  ( 7.097632634466814139, -2.668286824980076855, 14.00000000000000000 ) ) ;
#1686=CARTESIAN_POINT ( 'NONE',  ( -10.17357856257854110, 2.902115915870757679, 1.999999999999998224 ) ) ;
#1687=CARTESIAN_POINT ( 'NONE',  ( 6.997680802075244344, 0.4609939245309428446, 13.99999999999999645 ) ) ;
#1690=CARTESIAN_POINT ( 'NONE',  ( -0.1241967792452471353, -7.777596356722545679, 1.999999999999998224 ) ) ;
#1691=CARTESIAN_POINT ( 'NONE',  ( -6.551010013419180211, 0.8677952034721564400, 1.999999999999998224 ) ) ;
#1692=CARTESIAN_POINT ( 'NONE',  ( -6.762100275670005267, 3.470635719505328787, 13.99999999999999645 ) ) ;
#1695=CARTESIAN_POINT ( 'NONE',  ( -4.983290658055095967, 7.721050520723657051, 1.999999999999998224 ) ) ;
#1700=ORIENTED_EDGE ( 'NONE', *, *, #5176, .F. ) ;
#1703=VECTOR ( 'NONE', #5157, 1000.000000000000000 ) ;
#1704=CARTESIAN_POINT ( 'NONE',  ( 3.158576809044846279, 9.313732666428190754, 13.99999999999999645 ) ) ;
#1712=CARTESIAN_POINT ( 'NONE',  ( 0.5385325299235224072, 8.270587056550175120, 14.00000000000000000 ) ) ;
#1713=CARTESIAN_POINT ( 'NONE',  ( 3.426039378954556902, 5.938690629332269211, 1.999999999999998224 ) ) ;
#1718=CARTESIAN_POINT ( 'NONE',  ( -5.581220830679986200, 5.949058968288507110, 14.00000000000000000 ) ) ;
#1722=CARTESIAN_POINT ( 'NONE',  ( 1.869626052002640648, 6.555486721476421863, 13.99999999999999645 ) ) ;
#1724=CARTESIAN_POINT ( 'NONE',  ( -6.681386044268610824, 6.252046474378027519, 1.999999999999998224 ) ) ;
#1725=CARTESIAN_POINT ( 'NONE',  ( 1.869626052002579808, 6.555486721476420087, 1.999999999999998224 ) ) ;
#1727=CARTESIAN_POINT ( 'NONE',  ( 3.747087600548785868, -7.295897990121166465, 13.99999999999999645 ) ) ;
#1729=SURFACE_STYLE_USAGE ( .BOTH. , #456 ) ;
#1735=CARTESIAN_POINT ( 'NONE',  ( -7.551678268146210016, 5.989845445213457964, 13.99999999999999645 ) ) ;
#1740=CARTESIAN_POINT ( 'NONE',  ( -6.700137237868793783, -5.881230172876196427, 14.00000000000000000 ) ) ;
#1741=CARTESIAN_POINT ( 'NONE',  ( -2.440069559021786905, 10.46881825416662259, 13.99999999999999645 ) ) ;
#1743=CARTESIAN_POINT ( 'NONE',  ( -6.667513054348625623, -4.302816426345352774, 14.00000000000000000 ) ) ;
#1746=CARTESIAN_POINT ( 'NONE',  ( 6.026041665150466464, -0.9817477132364120784, 13.99999999999999645 ) ) ;
#1748=CARTESIAN_POINT ( 'NONE',  ( 8.549805251451806143, -4.382211019330641832, 1.999999999999998224 ) ) ;
#1749=CARTESIAN_POINT ( 'NONE',  ( 3.426039378954556902, 5.938690629332269211, 1.999999999999998224 ) ) ;
#1752=CARTESIAN_POINT ( 'NONE',  ( 5.500000000000000000, 0.000000000000000000, 1.999999999999998224 ) ) ;
#1753=CARTESIAN_POINT ( 'NONE',  ( -2.744490807750914030, 5.556819979548925481, 1.999999999999998224 ) ) ;
#1757=CARTESIAN_POINT ( 'NONE',  ( 10.98697916625460991, 0.8999353979983718554, 13.99999999999999645 ) ) ;
#1763=CARTESIAN_POINT ( 'NONE',  ( -3.391372024942433949, 7.476497417048839189, 14.00000000000000000 ) ) ;
#1764=CARTESIAN_POINT ( 'NONE',  ( 6.997680802075242568, 0.4609939245310665235, 1.999999999999998224 ) ) ;
#1767=CARTESIAN_POINT ( 'NONE',  ( 7.716263785693138644, -3.801003699433110228, 14.00000000000000000 ) ) ;
#1770=CARTESIAN_POINT ( 'NONE',  ( 4.476660083460862971, 9.887553134099890784, 1.999999999999998224 ) ) ;
#1773=CARTESIAN_POINT ( 'NONE',  ( 5.194219494279654015, 4.554949839096549269, 13.99999999999999645 ) ) ;
#1775=CARTESIAN_POINT ( 'NONE',  ( -0.7616497023963333390, 9.236585841460744462, 1.999999999999998224 ) ) ;
#1776=CARTESIAN_POINT ( 'NONE',  ( 6.444084565535371567, 4.617298776321547393, 1.999999999999998224 ) ) ;
#1779=CARTESIAN_POINT ( 'NONE',  ( 10.48651993945612126, 0.8648464362367445091, 1.999999999999998224 ) ) ;
#1784=DIRECTION ( 'NONE',  ( 0.9999273757268464236, -0.01205169166640770832, 0.000000000000000000 ) ) ;
#1786=CARTESIAN_POINT ( 'NONE',  ( 4.476660083460862971, 9.887553134100658170, 13.99999999999999645 ) ) ;
#1793=CARTESIAN_POINT ( 'NONE',  ( -8.757712506721391676, -2.046213373001789737, 14.00000000000000000 ) ) ;
#1794=CARTESIAN_POINT ( 'NONE',  ( -1.189470317277863121, -7.202885406307536265, 1.999999999999998224 ) ) ;
#1798=CARTESIAN_POINT ( 'NONE',  ( 3.520917041835319505, -6.848083076131263880, 14.00000000000000000 ) ) ;
#1800=CARTESIAN_POINT ( 'NONE',  ( 1.176163838800080574, -10.19826953922189539, 1.999999999999998224 ) ) ;
#1803=CARTESIAN_POINT ( 'NONE',  ( 6.938542625487071902, -1.260128425111980643, 13.99999999999999645 ) ) ;
#1804=CARTESIAN_POINT ( 'NONE',  ( -8.913799778910963312, 1.613954699392611047, 1.999999999999998224 ) ) ;
#1805=CARTESIAN_POINT ( 'NONE',  ( 1.183015137239217474, -7.150809911821259135, 1.999999999999998224 ) ) ;
#1811=CARTESIAN_POINT ( 'NONE',  ( -0.3669926094919909731, -5.824518274481597757, 1.999999999999998224 ) ) ;
#1816=DIRECTION ( 'NONE',  ( 1.445602896647339163E-16, 0.000000000000000000, 1.000000000000000000 ) ) ;
#1819=CARTESIAN_POINT ( 'NONE',  ( -4.581738566658776435, -9.288989786611782762, 13.99999999999999645 ) ) ;
#1824=CARTESIAN_POINT ( 'NONE',  ( 5.071900148311402567, 7.881338450277072027, 14.00000000000000000 ) ) ;
#1825=CARTESIAN_POINT ( 'NONE',  ( -5.810612947751084612, -4.611264106266946605, 1.999999999999998224 ) ) ;
#1826=CARTESIAN_POINT ( 'NONE',  ( -2.138212235155099616, 7.953261502403489835, 1.999999999999998224 ) ) ;
#1827=CARTESIAN_POINT ( 'NONE',  ( 8.618507686539667034, 3.909830026712121764, 14.00000000000000000 ) ) ;
#1829=CARTESIAN_POINT ( 'NONE',  ( -10.48421140591450751, 1.206973991593908169, 1.999999999999998224 ) ) ;
#1831=CARTESIAN_POINT ( 'NONE',  ( -0.1462562576243747192, 8.775315755192165668, 13.99999999999999645 ) ) ;
#1832=CARTESIAN_POINT ( 'NONE',  ( -5.745624475482375537, 5.035517847229356470, 13.99999999999999645 ) ) ;
#1834=CARTESIAN_POINT ( 'NONE',  ( -8.290222237438479524, 3.747600907060152142, 1.999999999999998224 ) ) ;
#1836=CARTESIAN_POINT ( 'NONE',  ( 6.938542625487070126, -1.260128425111949557, 1.999999999999998224 ) ) ;
#1840=CARTESIAN_POINT ( 'NONE',  ( 1.492118473828444536, -5.588909376072070501, 1.999999999999998224 ) ) ;
#1845=CARTESIAN_POINT ( 'NONE',  ( 7.066195124645641812, -7.302433507960033765, 13.99999999999999645 ) ) ;
#1850=CARTESIAN_POINT ( 'NONE',  ( -4.668631340267771712, 9.078485505802326827, 14.00000000000000000 ) ) ;
#1851=CARTESIAN_POINT ( 'NONE',  ( 7.812003909081975728, 1.689803927524521354, 1.999999999999998224 ) ) ;
#1852=ADVANCED_BREP_SHAPE_REPRESENTATION ( '', ( #2585, #1336 ), #2498 ) ;
#1853=CARTESIAN_POINT ( 'NONE',  ( -3.391372024942433505, 7.476497417048837413, 1.999999999999998224 ) ) ;
#1854=CARTESIAN_POINT ( 'NONE',  ( -8.999716648909560135, -0.5976852874978595409, 14.00000000000000000 ) ) ;
#1856=CARTESIAN_POINT ( 'NONE',  ( 7.775655769254118610, 6.170250810330676572, 1.999999999999998224 ) ) ;
#1858=CARTESIAN_POINT ( 'NONE',  ( 6.401046915552173644, 6.194151307163302533, 13.99999999999999645 ) ) ;
#1860=CARTESIAN_POINT ( 'NONE',  ( -8.486979168634645632, -0.6954046021538184963, 13.99999999999999645 ) ) ;
#1861=CARTESIAN_POINT ( 'NONE',  ( -8.332455577110955858, 5.761155596213678010, 1.999999999999998224 ) ) ;
#1862=CARTESIAN_POINT ( 'NONE',  ( 5.862282306371745300, 6.688714470717011196, 1.999999999999998224 ) ) ;
#1865=CARTESIAN_POINT ( 'NONE',  ( -6.069783318623453106, -0.2142533344232669390, 1.999999999999998224 ) ) ;
#1871=CARTESIAN_POINT ( 'NONE',  ( -9.913420430684192652, 3.732070475089104722, 13.99999999999999645 ) ) ;
#1878=CARTESIAN_POINT ( 'NONE',  ( -8.913799778910966864, 1.613954699392568859, 14.00000000000000000 ) ) ;
#1879=CARTESIAN_POINT ( 'NONE',  ( 1.649120185255090298, 7.633850905136056575, 1.999999999999998224 ) ) ;
#1881=CARTESIAN_POINT ( 'NONE',  ( 8.156937663705429387, 2.333191796391003603, 1.999999999999998224 ) ) ;
#1882=CARTESIAN_POINT ( 'NONE',  ( -0.7616497023963333390, 9.236585841461440793, 14.00000000000000000 ) ) ;
#1885=CARTESIAN_POINT ( 'NONE',  ( 1.933011552319068960, 10.64041406927699640, 1.999999999999998224 ) ) ;
#1886=CARTESIAN_POINT ( 'NONE',  ( 1.492118473828444536, -5.588909376072072277, 14.00000000000000000 ) ) ;
#1887=CARTESIAN_POINT ( 'NONE',  ( 5.857810772706378621, -5.665644577056677456, 13.99999999999999645 ) ) ;
#1888=EDGE_CURVE ( 'NONE', #3442, #660, #1095, .T. ) ;
#1890=CARTESIAN_POINT ( 'NONE',  ( 0.7175617537426050019, 6.248173425771539335, 14.00000000000000000 ) ) ;
#1893=CARTESIAN_POINT ( 'NONE',  ( 7.565999024956892249, -2.848076369834589450, 1.999999999999998224 ) ) ;
#1896=CARTESIAN_POINT ( 'NONE',  ( -7.019001384594680815, 0.4577903460188660345, 1.999999999999998224 ) ) ;
#1898=CARTESIAN_POINT ( 'NONE',  ( 6.034497645749723027, 4.327592090611793729, 1.999999999999998224 ) ) ;
#1908=CARTESIAN_POINT ( 'NONE',  ( -2.331745755519268215, 9.978964459600446091, 14.00000000000000000 ) ) ;
#1909=CARTESIAN_POINT ( 'NONE',  ( -3.441860715206332078, -7.602597312514155270, 1.999999999999998224 ) ) ;
#1912=CARTESIAN_POINT ( 'NONE',  ( 6.037635170864973588, 5.848285684830694997, 1.999999999999998224 ) ) ;
#1913=CARTESIAN_POINT ( 'NONE',  ( 8.256732931686221022, 4.597988481711512421, 14.00000000000000000 ) ) ;
#1914=EDGE_LOOP ( 'NONE', ( #5160, #1991, #895, #440 ) ) ;
#1917=CARTESIAN_POINT ( 'NONE',  ( -8.126042061586270293, 2.755650963504471473, 13.99999999999999645 ) ) ;
#1918=CARTESIAN_POINT ( 'NONE',  ( -2.331745755519268215, 9.978964459600444314, 1.999999999999998224 ) ) ;
#1920=CARTESIAN_POINT ( 'NONE',  ( 1.954797901281672967, -9.037865403626939909, 1.999999999999998224 ) ) ;
#1922=CARTESIAN_POINT ( 'NONE',  ( -4.975175822334872322, 5.137265612443480123, 1.999999999999998224 ) ) ;
#1924=CARTESIAN_POINT ( 'NONE',  ( 2.690160903457118557, 6.823041841979407884, 1.999999999999998224 ) ) ;
#1933=CARTESIAN_POINT ( 'NONE',  ( -3.672794075660814617, 8.451992513476522362, 14.00000000000000000 ) ) ;
#1934=CARTESIAN_POINT ( 'NONE',  ( 8.396466517619506575, 3.163083589105210258, 1.999999999999998224 ) ) ;
#1936=CARTESIAN_POINT ( 'NONE',  ( 1.881113203117336097, 8.098457488329447784, 1.999999999999998224 ) ) ;
#1937=CARTESIAN_POINT ( 'NONE',  ( 0.3244988297792451570, -9.772062696132405080, 14.00000000000000000 ) ) ;
#1941=CARTESIAN_POINT ( 'NONE',  ( 4.815977876496241095, 4.225366587634054483, 14.00000000000000000 ) ) ;
#1942=CARTESIAN_POINT ( 'NONE',  ( 10.02932042447482353, 0.1670047327946668492, 13.99999999999999645 ) ) ;
#1944=CARTESIAN_POINT ( 'NONE',  ( 10.50003631213657762, 0.006025845833179020727, 1.999999999999998224 ) ) ;
#1945=ORIENTED_EDGE ( 'NONE', *, *, #2908, .F. ) ;
#1946=CARTESIAN_POINT ( 'NONE',  ( 7.761517335261689965, -2.213789340049559407, 1.999999999999998224 ) ) ;
#1948=CARTESIAN_POINT ( 'NONE',  ( -0.2403693791186040096, 7.265099133626553574, 1.999999999999998224 ) ) ;
#1951=CARTESIAN_POINT ( 'NONE',  ( 7.494325059173603698, -0.8592991332473469690, 1.999999999999998224 ) ) ;
#1961=CARTESIAN_POINT ( 'NONE',  ( 9.020117466466054168, 0.2947087185667776055, 1.999999999999998224 ) ) ;
#1962=CARTESIAN_POINT ( 'NONE',  ( 6.033242055734853615, 5.122103984031451063, 13.99999999999999645 ) ) ;
#1963=CARTESIAN_POINT ( 'NONE',  ( 1.837295235934470305, 10.14794156482770049, 1.999999999999998224 ) ) ;
#1971=CARTESIAN_POINT ( 'NONE',  ( -2.189112655477411185, -6.464091385745795115, 14.00000000000000000 ) ) ;
#1972=CARTESIAN_POINT ( 'NONE',  ( -7.044187934146358465, 6.598551529630926282, 13.99999999999999645 ) ) ;
#1975=CARTESIAN_POINT ( 'NONE',  ( -6.398096652174580790, -7.548242073784104278, 1.999999999999998224 ) ) ;
#1977=CARTESIAN_POINT ( 'NONE',  ( -3.441860715206332078, -7.602597312514155270, 1.999999999999998224 ) ) ;
#1980=CARTESIAN_POINT ( 'NONE',  ( -4.184906021401388898, -5.457255036755482180, 1.999999999999998224 ) ) ;
#1984=CARTESIAN_POINT ( 'NONE',  ( 6.445330636073144603, -1.168293168414208827, 1.999999999999998224 ) ) ;
#1991=ORIENTED_EDGE ( 'NONE', *, *, #3567, .T. ) ;
#1994=CARTESIAN_POINT ( 'NONE',  ( -8.026550172065139321, -2.724140490265046122, 1.999999999999998224 ) ) ;
#1997=CARTESIAN_POINT ( 'NONE',  ( -5.390757458300978300, 6.793134358447313836, 13.99999999999999645 ) ) ;
#2002=VERTEX_POINT ( 'NONE', #3558 ) ;
#2005=CARTESIAN_POINT ( 'NONE',  ( 4.290186206382709422, 5.996800006796702220, 14.00000000000000000 ) ) ;
#2006=CARTESIAN_POINT ( 'NONE',  ( 5.348203032363755050, 8.300083771889282147, 13.99999999999999645 ) ) ;
#2007=CARTESIAN_POINT ( 'NONE',  ( -2.717942380035140992, -6.274577315194989957, 14.00000000000000000 ) ) ;
#2010=CARTESIAN_POINT ( 'NONE',  ( -8.402144917908874078, 4.670158400850170644, 1.999999999999998224 ) ) ;
#2012=CARTESIAN_POINT ( 'NONE',  ( -7.945923533235636604, 1.308497053349305439, 1.999999999999998224 ) ) ;
#2014=CARTESIAN_POINT ( 'NONE',  ( -6.334648143026943679, -2.872559841353752308, 1.999999999999998224 ) ) ;
#2015=CARTESIAN_POINT ( 'NONE',  ( -1.424809953814531127, 6.586142414399820844, 1.999999999999998224 ) ) ;
#2016=CARTESIAN_POINT ( 'NONE',  ( 2.321214644803172522, -6.838859567843808662, 13.99999999999999645 ) ) ;
#2022=CARTESIAN_POINT ( 'NONE',  ( 10.48651993945768623, 0.8648464362367445091, 14.00000000000000000 ) ) ;
#2023=CARTESIAN_POINT ( 'NONE',  ( 4.326322805049506393, -6.952463250691141461, 1.999999999999998224 ) ) ;
#2024=CARTESIAN_POINT ( 'NONE',  ( -6.465640026559317022, 4.020973141382162552, 13.99999999999999645 ) ) ;
#2030=CARTESIAN_POINT ( 'NONE',  ( -0.8347742375825083494, 7.207659102801796891, 14.00000000000000000 ) ) ;
#2031=CARTESIAN_POINT ( 'NONE',  ( 7.066195124645641812, -7.302433507960033765, 13.99999999999999645 ) ) ;
#2033=CARTESIAN_POINT ( 'NONE',  ( 6.315449825284095375, 1.474116854620425299, 14.00000000000000000 ) ) ;
#2035=CARTESIAN_POINT ( 'NONE',  ( 5.348203032363056053, 8.300083771889280371, 1.999999999999998224 ) ) ;
#2037=CARTESIAN_POINT ( 'NONE',  ( -0.1423371034015438186, 8.273642750285960190, 1.999999999999998224 ) ) ;
#2039=CARTESIAN_POINT ( 'NONE',  ( -6.792624376349764681, -3.077375260545992752, 13.99999999999999645 ) ) ;
#2046=CARTESIAN_POINT ( 'NONE',  ( 1.837295235934470528, 10.14794156482770404, 14.00000000000000000 ) ) ;
#2047=CARTESIAN_POINT ( 'NONE',  ( -8.411612136543093143, -4.319922787977411360, 1.999999999999998224 ) ) ;
#2048=CARTESIAN_POINT ( 'NONE',  ( 7.344045208303976224, 5.086154276871550195, 13.99999999999999645 ) ) ;
#2049=CARTESIAN_POINT ( 'NONE',  ( -3.139313036748870189, 9.741172307225710369, 14.00000000000000000 ) ) ;
#2054=CARTESIAN_POINT ( 'NONE',  ( 6.941605245898609056, 2.746080019685927187, 14.00000000000000000 ) ) ;
#2055=CARTESIAN_POINT ( 'NONE',  ( 3.158576809044846279, 9.313732666428190754, 13.99999999999999645 ) ) ;
#2057=CARTESIAN_POINT ( 'NONE',  ( 0.5542950790998155686, -6.736796398737816105, 14.00000000000000000 ) ) ;
#2060=CARTESIAN_POINT ( 'NONE',  ( -6.537688394901212341, -6.759197365500154930, 1.999999999999998224 ) ) ;
#2066=CARTESIAN_POINT ( 'NONE',  ( 2.690160903457118557, 6.823041841979407884, 1.999999999999998224 ) ) ;
#2070=CARTESIAN_POINT ( 'NONE',  ( -7.521311085815508335, -0.1255077825093697530, 13.99999999999999645 ) ) ;
#2073=CARTESIAN_POINT ( 'NONE',  ( 5.710084532570392390, 7.448680193042510389, 1.999999999999998224 ) ) ;
#2077=AXIS2_PLACEMENT_3D ( 'NONE', #5177, #5670, #5555 ) ;
#2080=CARTESIAN_POINT ( 'NONE',  ( 4.074896204546096357, -8.256886768010264888, 13.99999999999999645 ) ) ;
#2087=CARTESIAN_POINT ( 'NONE',  ( 1.103627080440590547, -6.655442145117441477, 14.00000000000000000 ) ) ;
#2088=CARTESIAN_POINT ( 'NONE',  ( 5.806279480217827249, -1.975834710110474512, 1.999999999999998224 ) ) ;
#2090=CARTESIAN_POINT ( 'NONE',  ( 3.622712361020366867, 5.236663886535375845, 14.00000000000000000 ) ) ;
#2093=CARTESIAN_POINT ( 'NONE',  ( -0.7976699882155984245, 9.736979168371712845, 1.999999999999998224 ) ) ;
#2095=CARTESIAN_POINT ( 'NONE',  ( -7.550296695603107899, -2.566425989403007257, 1.999999999999998224 ) ) ;
#2097=CARTESIAN_POINT ( 'NONE',  ( -4.492165532403490147, -5.853844512260857336, 13.99999999999999645 ) ) ;
#2099=CARTESIAN_POINT ( 'NONE',  ( -9.926332099420363875, -1.311590842189569894, 1.999999999999998224 ) ) ;
#2102=APPLICATION_CONTEXT ( 'automotive_design' ) ;
#2106=CARTESIAN_POINT ( 'NONE',  ( -9.247353065532886163, -2.155497948345618919, 13.99999999999999645 ) ) ;
#2112=CARTESIAN_POINT ( 'NONE',  ( 8.370269057508139099, -1.803949267857856142, 14.00000000000000000 ) ) ;
#2113=CARTESIAN_POINT ( 'NONE',  ( -9.913420430684192652, 3.732070475089104722, 13.99999999999999645 ) ) ;
#2116=FACE_OUTER_BOUND ( 'NONE', #1914, .T. ) ;
#2117=CARTESIAN_POINT ( 'NONE',  ( 6.004028658818958419, -2.715480180205860794, 14.00000000000000000 ) ) ;
#2120=CARTESIAN_POINT ( 'NONE',  ( 1.933011552319068960, 10.64041406927699640, 1.999999999999998224 ) ) ;
#2122=CARTESIAN_POINT ( 'NONE',  ( 6.638644669766899931, 2.135480210976827831, 13.99999999999999645 ) ) ;
#2124=CARTESIAN_POINT ( 'NONE',  ( -4.895455514773497718, -6.178604150901914061, 1.999999999999998224 ) ) ;
#2126=CARTESIAN_POINT ( 'NONE',  ( -5.402835942920536816, -5.063607225391134392, 13.99999999999999645 ) ) ;
#2128=CARTESIAN_POINT ( 'NONE',  ( 2.678407690932628871, -9.362678857629568085, 1.999999999999998224 ) ) ;
#2136=CARTESIAN_POINT ( 'NONE',  ( 0.7976699882155482424, 9.763020831628288931, 13.99999999999999645 ) ) ;
#2142=CARTESIAN_POINT ( 'NONE',  ( -7.892574838092353495, -1.309761382309196032, 14.00000000000000000 ) ) ;
#2143=CARTESIAN_POINT ( 'NONE',  ( 2.406079317367887160, 6.392288322179701332, 1.999999999999998224 ) ) ;
#2146=CARTESIAN_POINT ( 'NONE',  ( 7.925371078819432036, 2.990572132494779378, 14.00000000000000000 ) ) ;
#2150=CARTESIAN_POINT ( 'NONE',  ( -1.189470317277863565, -7.202885406307538041, 13.99999999999999645 ) ) ;
#2153=CARTESIAN_POINT ( 'NONE',  ( -5.048038583874033591, -7.300734008993713609, 1.999999999999998224 ) ) ;
#2154=CARTESIAN_POINT ( 'NONE',  ( 6.033242055734851839, 5.122103984031729063, 1.999999999999998224 ) ) ;
#2155=CARTESIAN_POINT ( 'NONE',  ( 6.679452517770527287, -4.623421500472437273, 13.99999999999999645 ) ) ;
#2158=CARTESIAN_POINT ( 'NONE',  ( -8.929154442179981999, -4.413097966322209409, 1.999999999999998224 ) ) ;
#2160=CARTESIAN_POINT ( 'NONE',  ( 5.500000000000000000, 0.000000000000000000, 1.999999999999998224 ) ) ;
#2165=CARTESIAN_POINT ( 'NONE',  ( 8.952336951391263398, 1.032601321559317276, 13.99999999999999645 ) ) ;
#2172=EDGE_CURVE ( 'NONE', #2002, #3473, #2406, .T. ) ;
#2173=CARTESIAN_POINT ( 'NONE',  ( -2.415560149437796511, -8.486491385245610530, 14.00000000000000000 ) ) ;
#2174=CARTESIAN_POINT ( 'NONE',  ( -0.7077576507784110182, 10.75210906117156995, 13.99999999999999645 ) ) ;
#2177=CARTESIAN_POINT ( 'NONE',  ( 0.5141566911144540564, -7.748312628312728378, 14.00000000000000000 ) ) ;
#2181=CARTESIAN_POINT ( 'NONE',  ( 6.180183843827204093, 3.174252413088802793, 13.99999999999999645 ) ) ;
#2183=CARTESIAN_POINT ( 'NONE',  ( -8.547479018124427341, -2.754496926847987748, 1.999999999999998224 ) ) ;
#2185=CARTESIAN_POINT ( 'NONE',  ( 5.586635445632133212, -4.430858740432559451, 1.999999999999998224 ) ) ;
#2190=CARTESIAN_POINT ( 'NONE',  ( -3.922355934210176809, -4.464780306276820099, 1.999999999999998224 ) ) ;
#2194=CARTESIAN_POINT ( 'NONE',  ( 1.176163838800443395, -10.19826953922044765, 13.99999999999999645 ) ) ;
#2202=CARTESIAN_POINT ( 'NONE',  ( -7.652305818843811558, 2.590529227167490234, 14.00000000000000000 ) ) ;
#2203=CARTESIAN_POINT ( 'NONE',  ( 10.98697916625460991, 0.8999353979983718554, 13.99999999999999645 ) ) ;
#2205=CARTESIAN_POINT ( 'NONE',  ( 2.543939756934300966, 7.929199913827024382, 14.00000000000000000 ) ) ;
#2207=CARTESIAN_POINT ( 'NONE',  ( 2.810994617404584783, -9.846529629019117991, 1.999999999999998224 ) ) ;
#2210=CARTESIAN_POINT ( 'NONE',  ( 7.025143070632195119, -0.1151745751371588272, 13.99999999999999645 ) ) ;
#2212=CARTESIAN_POINT ( 'NONE',  ( -4.983290658055095967, 7.721050520723657051, 1.999999999999998224 ) ) ;
#2213=CARTESIAN_POINT ( 'NONE',  ( -7.364573508975982286, 1.714675912027187943, 1.999999999999998224 ) ) ;
#2215=FILL_AREA_STYLE_COLOUR ( '', #3606 ) ;
#2217=CARTESIAN_POINT ( 'NONE',  ( 4.443413384189978110, 4.597174039215664365, 1.999999999999998224 ) ) ;
#2221=CARTESIAN_POINT ( 'NONE',  ( -10.53467355220997526, 0.3418899515811328338, 13.99999999999999645 ) ) ;
#2225=CARTESIAN_POINT ( 'NONE',  ( 7.017208779832877497, -5.019401656905778886, 14.00000000000000000 ) ) ;
#2226=CARTESIAN_POINT ( 'NONE',  ( 4.585040342817966241, 6.402697129001492904, 1.999999999999998224 ) ) ;
#2229=CARTESIAN_POINT ( 'NONE',  ( -0.2798806129217078498, -8.779921314117062892, 14.00000000000000000 ) ) ;
#2231=CARTESIAN_POINT ( 'NONE',  ( 5.279590631141700463, 9.498297537454860162, 1.999999999999998224 ) ) ;
#2233=CARTESIAN_POINT ( 'NONE',  ( 4.914575889516433094, -3.754581871930561032, 13.99999999999999645 ) ) ;
#2234=CARTESIAN_POINT ( 'NONE',  ( -3.672794075660469559, 8.451992513476518809, 1.999999999999998224 ) ) ;
#2236=CARTESIAN_POINT ( 'NONE',  ( -2.721086536275891810, 7.222755814214461445, 1.999999999999998224 ) ) ;
#2238=UNCERTAINTY_MEASURE_WITH_UNIT (LENGTH_MEASURE( 1.000000000000000082E-05 ), #397, 'distance_accuracy_value', 'NONE');
#2241=CARTESIAN_POINT ( 'NONE',  ( 1.492118473828444536, -5.588909376072070501, 1.999999999999998224 ) ) ;
#2253=CARTESIAN_POINT ( 'NONE',  ( 8.256732931686221022, 4.597988481711512421, 14.00000000000000000 ) ) ;
#2254=CARTESIAN_POINT ( 'NONE',  ( 7.565999024956892249, -2.848076369834589450, 1.999999999999998224 ) ) ;
#2256=CARTESIAN_POINT ( 'NONE',  ( -8.013356705133178437, 0.6503825268544296545, 1.999999999999998224 ) ) ;
#2257=CARTESIAN_POINT ( 'NONE',  ( -1.480145937554535385, 8.115026467927430431, 14.00000000000000000 ) ) ;
#2259=CARTESIAN_POINT ( 'NONE',  ( -9.742306995815773973, -3.848972158781406083, 1.999999999999998224 ) ) ;
#2260=CARTESIAN_POINT ( 'NONE',  ( 5.460516619045268527, 3.400499599735717915, 14.00000000000000000 ) ) ;
#2261=CARTESIAN_POINT ( 'NONE',  ( -7.245889760505164645, 4.668767092638694827, 13.99999999999999645 ) ) ;
#2263=CARTESIAN_POINT ( 'NONE',  ( 4.585040342817689130, 6.402697129001494680, 13.99999999999999645 ) ) ;
#2264=CARTESIAN_POINT ( 'NONE',  ( 7.017208779832875720, -5.019401656906101294, 1.999999999999998224 ) ) ;
#2267=CARTESIAN_POINT ( 'NONE',  ( -7.519441789400336695, 0.4931591957933217363, 1.999999999999998224 ) ) ;
#2270=CARTESIAN_POINT ( 'NONE',  ( -5.183646570197097958, -3.010418922387011698, 1.999999999999998224 ) ) ;
#2274=DIRECTION ( 'NONE',  ( -0.01205169166640770832, -0.9999273757268464236, -2.258590485605784177E-18 ) ) ;
#2275=CARTESIAN_POINT ( 'NONE',  ( 7.631804465920718705, -6.689046765414282447, 13.99999999999999645 ) ) ;
#2280=CARTESIAN_POINT ( 'NONE',  ( 8.549805251451807919, -4.382211019330642721, 14.00000000000000000 ) ) ;
#2281=CARTESIAN_POINT ( 'NONE',  ( 4.793600759081159346, 4.956424179878264447, 1.999999999999998224 ) ) ;
#2282=CARTESIAN_POINT ( 'NONE',  ( -6.185289998984973003, -6.402116997106289453, 1.999999999999998224 ) ) ;
#2283=CARTESIAN_POINT ( 'NONE',  ( -6.700137237868793783, -5.881230172876196427, 14.00000000000000000 ) ) ;
#2285=CARTESIAN_POINT ( 'NONE',  ( 3.158576809044846279, 9.313732666428188978, 1.999999999999998224 ) ) ;
#2287=CARTESIAN_POINT ( 'NONE',  ( 2.701324588234351953, 8.405562337868641265, 13.99999999999999645 ) ) ;
#2289=CARTESIAN_POINT ( 'NONE',  ( -7.091148812992124739, -4.571561645351811976, 13.99999999999999645 ) ) ;
#2290=CARTESIAN_POINT ( 'NONE',  ( -6.048456868091351524, 0.8014113234714785872, 14.00000000000000000 ) ) ;
#2291=CARTESIAN_POINT ( 'NONE',  ( 1.870926337630253622, -8.025887876971653512, 1.999999999999998224 ) ) ;
#2295=CARTESIAN_POINT ( 'NONE',  ( 6.315449825284093599, 1.474116854620456163, 1.999999999999998224 ) ) ;
#2297=CARTESIAN_POINT ( 'NONE',  ( -0.3669926094919909731, -5.824518274481597757, 1.999999999999998224 ) ) ;
#2302=CARTESIAN_POINT ( 'NONE',  ( 8.671201137382265500, 6.657490096169393468, 13.99999999999999645 ) ) ;
#2308=CARTESIAN_POINT ( 'NONE',  ( 5.519166806814065573, -7.959527472086049826, 14.00000000000000000 ) ) ;
#2309=CARTESIAN_POINT ( 'NONE',  ( 4.366464973618271905, -5.686602709308029802, 1.999999999999998224 ) ) ;
#2310=CARTESIAN_POINT ( 'NONE',  ( -5.581220830680290845, 5.949058968288200688, 1.999999999999998224 ) ) ;
#2311=CARTESIAN_POINT ( 'NONE',  ( -4.354965481614498479, -8.841480220785717492, 14.00000000000000000 ) ) ;
#2313=CARTESIAN_POINT ( 'NONE',  ( 3.917689075872947235, 9.035181080458078995, 1.999999999999998224 ) ) ;
#2315=CARTESIAN_POINT ( 'NONE',  ( -4.060726170632903198, -7.305992298388080286, 13.99999999999999645 ) ) ;
#2317=CARTESIAN_POINT ( 'NONE',  ( 4.264126983937991611, 9.433107915010285893, 1.999999999999998224 ) ) ;
#2319=PRODUCT_DEFINITION_FORMATION_WITH_SPECIFIED_SOURCE ( 'ANY', '', #5046, .NOT_KNOWN. ) ;
#2320=CARTESIAN_POINT ( 'NONE',  ( 7.422282976138727228, -5.315384720684046549, 1.999999999999998224 ) ) ;
#2322=CARTESIAN_POINT ( 'NONE',  ( -3.715337444063474770, -5.771435016728991840, 1.999999999999998224 ) ) ;
#2324=CARTESIAN_POINT ( 'NONE',  ( 5.648567055624510225, 4.800053419556092216, 1.999999999999998224 ) ) ;
#2326=CARTESIAN_POINT ( 'NONE',  ( -6.551010013419181988, 0.8677952034721571062, 13.99999999999999645 ) ) ;
#2333=CARTESIAN_POINT ( 'NONE',  ( -1.515482495401828000, 9.129776367295956874, 14.00000000000000000 ) ) ;
#2334=CARTESIAN_POINT ( 'NONE',  ( 5.887534416617370425, 3.663839002572738313, 1.999999999999998224 ) ) ;
#2336=CARTESIAN_POINT ( 'NONE',  ( -7.966005157978614193, 4.422220743486963812, 1.999999999999998224 ) ) ;
#2337=CARTESIAN_POINT ( 'NONE',  ( -7.963215149404076598, -4.094909132697305054, 14.00000000000000000 ) ) ;
#2341=CARTESIAN_POINT ( 'NONE',  ( 0.2014543481397604030, 6.272771216426900942, 14.00000000000000000 ) ) ;
#2342=CARTESIAN_POINT ( 'NONE',  ( -7.884571930971329579, 3.418633173532294123, 13.99999999999999645 ) ) ;
#2344=CARTESIAN_POINT ( 'NONE',  ( -9.986481889893736863, 1.144076113142370899, 1.999999999999998224 ) ) ;
#2347=CARTESIAN_POINT ( 'NONE',  ( 4.074896204546095468, -8.256886768008961042, 1.999999999999998224 ) ) ;
#2350=CARTESIAN_POINT ( 'NONE',  ( -5.370374743918785221, 4.702532619530842339, 1.999999999999998224 ) ) ;
#2351=EDGE_LOOP ( 'NONE', ( #2443, #4417, #950, #4511 ) ) ;
#2352=CARTESIAN_POINT ( 'NONE',  ( -6.317162512443194267, 3.238855812894541941, 1.999999999999998224 ) ) ;
#2364=CARTESIAN_POINT ( 'NONE',  ( 2.992331685656917539, 8.840389773664524498, 14.00000000000000000 ) ) ;
#2365=CARTESIAN_POINT ( 'NONE',  ( 2.701324588234195190, 8.405562337868014211, 1.999999999999998224 ) ) ;
#2367=EDGE_CURVE ( 'NONE', #3324, #3442, #4885, .T. ) ;
#2368=B_SPLINE_CURVE_WITH_KNOTS ( 'NONE', 3,
 ( #5269, #3142, #3571, #2703, #2623, #3086, #1840, #2297, #4377, #3116, #2190, #3943, #1324, #2740, #979, #1, #483, #4457, #518, #1753, #4833, #4030, #5351, #1409, #4919, #892, #4402, #3538, #458, #2217, #2676, #3968, #1358, #4863, #4428, #690, #1089, #1984, #4602, #4120, #3310, #1006, #568, #5060, #3704, #3680, #5435, #3737, #2875, #2384, #2444, #603, #1029, #3202, #4087, #4999, #255, #4204, #2014, #1469, #1118, #1490, #2787, #2765, #4517, #2352, #198, #4628, #172, #3281, #140, #5465, #4573, #1060, #4971, #5522, #633, #1924, #2850, #4949, #3768, #2324, #1898, #3657, #4543, #5410, #3225, #4143, #1951, #1522, #3251, #5034, #661, #2821, #2412, #4173, #228, #5496, #1557, #2905, #4658, #1580, #3339, #5091, #1147, #2802, #4441, #4013, #3211, #3127, #70, #2369, #615, #2256, #3639, #3667, #3182, #1455, #497, #2310, #4554, #4042, #1853, #1826, #183, #4981, #2719, #1936, #5395, #991, #156, #4932, #1912, #1372, #4876, #583, #1881, #3584, #2686, #4129, #5337, #5421, #3155, #1477, #3609, #97, #932, #1395, #4901, #4102, #5365, #961, #4471, #1422, #3690, #2774, #531, #2282, #4959, #3234, #4528, #2750, #4502, #1041, #555, #4070, #122, #1016, #2336, #5214, #3029, #1644, #1695, #1073, #3264, #1212, #2998, #1501, #4712, #776, #2835, #4774, #2073, #1269, #3400, #5043, #4587, #3295, #807, #5446, #2499, #1538, #5583, #835, #5153, #1184, #2964, #2528, #3830, #5175, #2128, #2587, #3451, #645, #210, #2935, #311, #1236, #4346, #4291, #399, #2158, #4687, #344, #2099, #4260, #5015, #3857, #5608, #2397, #369, #747, #3718, #4156, #1669, #5478, #3424, #4743, #2560, #1963, #3884, #4320, #5636, #1323, #3084, #4487, #3996, #4029, #1384, #5324, #1779, #4455 ),
 .UNSPECIFIED., .F., .F.,
 ( 4, 2, 2, 2, 2, 2, 2, 2, 2, 2, 2, 2, 2, 2, 2, 2, 2, 2, 2, 2, 2, 2, 2, 2, 2, 2, 2, 2, 2, 2, 2, 2, 2, 2, 2, 2, 2, 2, 2, 2, 2, 2, 2, 2, 2, 2, 2, 2, 2, 2, 2, 2, 2, 2, 2, 2, 2, 2, 2, 2, 2, 2, 2, 2, 2, 2, 2, 2, 2, 2, 2, 2, 2, 2, 2, 2, 2, 2, 2, 2, 2, 2, 2, 2, 2, 2, 2, 2, 2, 2, 2, 2, 2, 2, 2, 2, 2, 2, 2, 2, 2, 2, 2, 2, 2, 2, 2, 2, 2, 2, 2, 2, 2, 2, 2, 2, 2, 2, 2, 2, 4 ),
 ( 0.000000000000000000, 0.01562500000000000000, 0.03125000000000000000, 0.04687500000000000000, 0.06250000000000000000, 0.07812500000000000000, 0.09375000000000000000, 0.1093750000000000000, 0.1250000000000000000, 0.1328125000000000000, 0.1406250000000000000, 0.1484375000000000000, 0.1562500000000000000, 0.1640625000000000000, 0.1718750000000000000, 0.1796875000000000000, 0.1875000000000000000, 0.1953125000000000000, 0.2031250000000000000, 0.2109375000000000000, 0.2187500000000000000, 0.2265625000000000000, 0.2343750000000000000, 0.2421875000000000000, 0.2500000000000000000, 0.2578125000000000000, 0.2656250000000000000, 0.2734375000000000000, 0.2812500000000000000, 0.2890625000000000000, 0.2968750000000000000, 0.3046875000000000000, 0.3125000000000000000, 0.3203125000000000000, 0.3281250000000000000, 0.3359375000000000000, 0.3437500000000000000, 0.3515625000000000000, 0.3593750000000000000, 0.3671875000000000000, 0.3750000000000000000, 0.3828125000000000000, 0.3906250000000000000, 0.3984375000000000000, 0.4062500000000000000, 0.4140625000000000000, 0.4218750000000000000, 0.4296875000000000000, 0.4375000000000000000, 0.4453125000000000000, 0.4531250000000000000, 0.4609375000000000000, 0.4687500000000000000, 0.4765625000000000000, 0.4843750000000000000, 0.4921875000000000000, 0.5000000000000000000, 0.5078125000000000000, 0.5156250000000000000, 0.5234375000000000000, 0.5312500000000000000, 0.5390625000000000000, 0.5468750000000000000, 0.5546875000000000000, 0.5625000000000000000, 0.5703125000000000000, 0.5781250000000000000, 0.5859375000000000000, 0.5937500000000000000, 0.6015625000000000000, 0.6093750000000000000, 0.6171875000000000000, 0.6250000000000000000, 0.6328125000000000000, 0.6406250000000000000, 0.6484375000000000000, 0.6562500000000000000, 0.6640625000000000000, 0.6718750000000000000, 0.6796875000000000000, 0.6875000000000000000, 0.6953125000000000000, 0.7031250000000000000, 0.7109375000000000000, 0.7187500000000000000, 0.7265625000000000000, 0.7343750000000000000, 0.7421875000000000000, 0.7500000000000000000, 0.7578125000000000000, 0.7656250000000000000, 0.7734375000000000000, 0.7812500000000000000, 0.7890625000000000000, 0.7968750000000000000, 0.8046875000000000000, 0.8125000000000000000, 0.8203125000000000000, 0.8281250000000000000, 0.8359375000000000000, 0.8437500000000000000, 0.8515625000000000000, 0.8593750000000000000, 0.8671875000000000000, 0.8750000000000000000, 0.8828125000000000000, 0.8906250000000000000, 0.8984375000000000000, 0.9062500000000000000, 0.9140625000000000000, 0.9218750000000000000, 0.9296875000000000000, 0.9375000000000000000, 0.9453125000000000000, 0.9531250000000000000, 0.9609375000000000000, 0.9687500000000000000, 0.9765625000000000000, 0.9843750000000000000, 0.9921875000000000000, 1.000000000000000000 ),
 .UNSPECIFIED. ) ;
#2369=CARTESIAN_POINT ( 'NONE',  ( -7.892574838092051515, -1.309761382309195366, 1.999999999999998224 ) ) ;
#2370=CARTESIAN_POINT ( 'NONE',  ( -8.763921109941536614, 2.343993041296470903, 14.00000000000000000 ) ) ;
#2373=CARTESIAN_POINT ( 'NONE',  ( 9.199536834907135585, 5.930433524309127513, 1.999999999999998224 ) ) ;
#2374=CARTESIAN_POINT ( 'NONE',  ( -3.595699629853522872, 5.016010494498949868, 14.00000000000000000 ) ) ;
#2375=CARTESIAN_POINT ( 'NONE',  ( -1.342170334697156742, -10.21728332006373030, 13.99999999999999645 ) ) ;
#2376=CARTESIAN_POINT ( 'NONE',  ( 9.602236826901936695, 4.172718697305983326, 1.999999999999998224 ) ) ;
#2378=CARTESIAN_POINT ( 'NONE',  ( 4.326322805049506393, -6.952463250691141461, 1.999999999999998224 ) ) ;
#2382=CARTESIAN_POINT ( 'NONE',  ( 4.848934754808810865, -4.539135254905419359, 1.999999999999998224 ) ) ;
#2384=CARTESIAN_POINT ( 'NONE',  ( -0.5497243705170606898, -6.763214047005217999, 1.999999999999998224 ) ) ;
#2394=CARTESIAN_POINT ( 'NONE',  ( 7.422282976138727228, -5.315384720684046549, 1.999999999999998224 ) ) ;
#2395=CARTESIAN_POINT ( 'NONE',  ( 1.015216742983949372, 7.730330528320555672, 13.99999999999999645 ) ) ;
#2397=CARTESIAN_POINT ( 'NONE',  ( -8.765969750979122566, 5.050798838973363125, 1.999999999999998224 ) ) ;
#2402=CARTESIAN_POINT ( 'NONE',  ( 4.848934754808812642, -4.539135254905673378, 14.00000000000000000 ) ) ;
#2403=CARTESIAN_POINT ( 'NONE',  ( -9.247353065532886163, -2.155497948345618919, 13.99999999999999645 ) ) ;
#2404=CARTESIAN_POINT ( 'NONE',  ( 0.1634456542307745064, 10.28566380800474533, 1.999999999999998224 ) ) ;
#2406=B_SPLINE_CURVE_WITH_KNOTS ( 'NONE', 3,
 ( #560, #4476, #188, #4533, #536, #1047, #1886, #5341, #966, #4559, #2778, #3643, #5400, #1459, #2840, #589, #621, #5426, #2374, #4963, #503, #1020, #3160, #2341, #4987, #4106, #4134, #3671, #1482, #2809, #1941, #2260, #4018, #75, #2724, #713, #3388, #4593, #650, #243, #4162, #1657, #2402, #5513, #736, #1629, #4276, #2087, #2464, #762, #216, #1971, #273, #2512, #3301, #296, #3412, #1199, #327, #3846, #2923, #5569, #5484, #5050, #2431, #5140, #3725, #1572, #677, #4646, #5597, #4221, #4192, #2030, #3785, #2893, #4245, #2948, #5541, #2005, #1546, #1108, #3757, #5076, #2054, #5164, #1596, #1225, #2865, #3328, #3357, #1168, #1134, #4618, #5112, #4675, #2490, #4701, #3813, #1681, #791, #1309, #1253, #3520, #845, #4306, #3436, #1337, #5254, #3013, #381, #2142, #3549, #3067, #3097, #2202, #4845, #2573, #467, #2601, #5228, #3896, #1763, #5653, #903, #4811, #1712, #3954, #4359, #2978, #4727, #415, #5280, #4786, #2660, #2543, #358, #13, #3494, #5621, #2112, #4758, #4412, #2225, #820, #3978, #1285, #3467, #3869, #5193, #4332, #38, #3040, #2173, #3928, #5682, #5309, #4389, #1740, #875, #2634, #444, #1793, #3125, #580, #1878, #4009, #2684, #4551, #66, #3635, #553, #5393, #1933, #5335, #2333, #611, #181, #5362, #2364, #494, #1824, #3607, #3688, #2772, #2253, #1370, #1451, #1475, #4526, #2748, #3209, #1014, #2280, #1418, #3152, #3665, #2308, #3582, #4929, #4127, #3232, #4439, #4873, #4499, #4978, #1393, #4099, #930, #5419, #1038, #2800, #4957, #152, #4899, #958, #2716, #4468, #4068, #527, #4040, #3179, #95, #988, #1850, #119, #1908, #3748, #5100, #2046, #5505, #5040, #3261, #5012, #4610, #2453, #1619, #2857, #5531, #642, #2022, #1099 ),
 .UNSPECIFIED., .F., .F.,
 ( 4, 2, 2, 2, 2, 2, 2, 2, 2, 2, 2, 2, 2, 2, 2, 2, 2, 2, 2, 2, 2, 2, 2, 2, 2, 2, 2, 2, 2, 2, 2, 2, 2, 2, 2, 2, 2, 2, 2, 2, 2, 2, 2, 2, 2, 2, 2, 2, 2, 2, 2, 2, 2, 2, 2, 2, 2, 2, 2, 2, 2, 2, 2, 2, 2, 2, 2, 2, 2, 2, 2, 2, 2, 2, 2, 2, 2, 2, 2, 2, 2, 2, 2, 2, 2, 2, 2, 2, 2, 2, 2, 2, 2, 2, 2, 2, 2, 2, 2, 2, 2, 2, 2, 2, 2, 2, 2, 2, 2, 2, 2, 2, 2, 2, 2, 2, 2, 2, 2, 2, 4 ),
 ( 0.000000000000000000, 0.01562500000000000000, 0.03125000000000000000, 0.04687500000000000000, 0.06250000000000000000, 0.07812500000000000000, 0.09375000000000000000, 0.1093750000000000000, 0.1250000000000000000, 0.1328125000000000000, 0.1406250000000000000, 0.1484375000000000000, 0.1562500000000000000, 0.1640625000000000000, 0.1718750000000000000, 0.1796875000000000000, 0.1875000000000000000, 0.1953125000000000000, 0.2031250000000000000, 0.2109375000000000000, 0.2187500000000000000, 0.2265625000000000000, 0.2343750000000000000, 0.2421875000000000000, 0.2500000000000000000, 0.2578125000000000000, 0.2656250000000000000, 0.2734375000000000000, 0.2812500000000000000, 0.2890625000000000000, 0.2968750000000000000, 0.3046875000000000000, 0.3125000000000000000, 0.3203125000000000000, 0.3281250000000000000, 0.3359375000000000000, 0.3437500000000000000, 0.3515625000000000000, 0.3593750000000000000, 0.3671875000000000000, 0.3750000000000000000, 0.3828125000000000000, 0.3906250000000000000, 0.3984375000000000000, 0.4062500000000000000, 0.4140625000000000000, 0.4218750000000000000, 0.4296875000000000000, 0.4375000000000000000, 0.4453125000000000000, 0.4531250000000000000, 0.4609375000000000000, 0.4687500000000000000, 0.4765625000000000000, 0.4843750000000000000, 0.4921875000000000000, 0.5000000000000000000, 0.5078125000000000000, 0.5156250000000000000, 0.5234375000000000000, 0.5312500000000000000, 0.5390625000000000000, 0.5468750000000000000, 0.5546875000000000000, 0.5625000000000000000, 0.5703125000000000000, 0.5781250000000000000, 0.5859375000000000000, 0.5937500000000000000, 0.6015625000000000000, 0.6093750000000000000, 0.6171875000000000000, 0.6250000000000000000, 0.6328125000000000000, 0.6406250000000000000, 0.6484375000000000000, 0.6562500000000000000, 0.6640625000000000000, 0.6718750000000000000, 0.6796875000000000000, 0.6875000000000000000, 0.6953125000000000000, 0.7031250000000000000, 0.7109375000000000000, 0.7187500000000000000, 0.7265625000000000000, 0.7343750000000000000, 0.7421875000000000000, 0.7500000000000000000, 0.7578125000000000000, 0.7656250000000000000, 0.7734375000000000000, 0.7812500000000000000, 0.7890625000000000000, 0.7968750000000000000, 0.8046875000000000000, 0.8125000000000000000, 0.8203125000000000000, 0.8281250000000000000, 0.8359375000000000000, 0.8437500000000000000, 0.8515625000000000000, 0.8593750000000000000, 0.8671875000000000000, 0.8750000000000000000, 0.8828125000000000000, 0.8906250000000000000, 0.8984375000000000000, 0.9062500000000000000, 0.9140625000000000000, 0.9218750000000000000, 0.9296875000000000000, 0.9375000000000000000, 0.9453125000000000000, 0.9531250000000000000, 0.9609375000000000000, 0.9687500000000000000, 0.9765625000000000000, 0.9843750000000000000, 0.9921875000000000000, 1.000000000000000000 ),
 .UNSPECIFIED. ) ;
#2407=CARTESIAN_POINT ( 'NONE',  ( -7.245889760505162869, 4.668767092638087313, 1.999999999999998224 ) ) ;
#2409=CARTESIAN_POINT ( 'NONE',  ( -6.317162512443194267, 3.238855812894541941, 1.999999999999998224 ) ) ;
#2412=CARTESIAN_POINT ( 'NONE',  ( 5.053476174607396842, -5.757900651972986950, 1.999999999999998224 ) ) ;
#2415=CARTESIAN_POINT ( 'NONE',  ( 9.320190601379009010, -2.164585516638707574, 1.999999999999998224 ) ) ;
#2421=CARTESIAN_POINT ( 'NONE',  ( 0.5754137710878161061, 8.770917875152035137, 1.999999999999998224 ) ) ;
#2423=CARTESIAN_POINT ( 'NONE',  ( -2.153669193480074018, -8.035861145135083206, 13.99999999999999645 ) ) ;
#2427=DIRECTION ( 'NONE',  ( -0.9999273757268464236, 0.01205169166640771006, 2.722181309742254022E-20 ) ) ;
#2431=CARTESIAN_POINT ( 'NONE',  ( -6.734745854536168252, 2.161492950162117399, 14.00000000000000000 ) ) ;
#2432=CARTESIAN_POINT ( 'NONE',  ( -8.411612136543094920, -4.319922787977579226, 13.99999999999999645 ) ) ;
#2434=CARTESIAN_POINT ( 'NONE',  ( 3.173694703385745886, 5.505084763670784476, 14.00000000000000000 ) ) ;
#2436=CARTESIAN_POINT ( 'NONE',  ( -1.592064345877699072, 9.625584969238365929, 1.999999999999998224 ) ) ;
#2440=CARTESIAN_POINT ( 'NONE',  ( 4.290186206382708534, 5.996800006796977556, 1.999999999999998224 ) ) ;
#2443=ORIENTED_EDGE ( 'NONE', *, *, #2367, .F. ) ;
#2444=CARTESIAN_POINT ( 'NONE',  ( -1.105557477332586247, -6.708264047591375956, 1.999999999999998224 ) ) ;
#2445=CARTESIAN_POINT ( 'NONE',  ( -2.965071238690785371, 6.007415411094349622, 1.999999999999998224 ) ) ;
#2446=CARTESIAN_POINT ( 'NONE',  ( -4.372214883940321428, 6.312905667202753257, 13.99999999999999645 ) ) ;
#2453=CARTESIAN_POINT ( 'NONE',  ( 8.269507991092027055, 6.356934974246627235, 14.00000000000000000 ) ) ;
#2454=CARTESIAN_POINT ( 'NONE',  ( -5.337360893037004672, -7.710592058383595848, 1.999999999999998224 ) ) ;
#2457=CARTESIAN_POINT ( 'NONE',  ( 6.679452517770527287, -4.623421500472437273, 13.99999999999999645 ) ) ;
#2464=CARTESIAN_POINT ( 'NONE',  ( 0.5542950790998155686, -6.736796398737816105, 14.00000000000000000 ) ) ;
#2465=CARTESIAN_POINT ( 'NONE',  ( 8.993528569561179964, -4.616306094804236260, 13.99999999999999645 ) ) ;
#2466=CARTESIAN_POINT ( 'NONE',  ( 2.690160903457257557, 6.823041841979409661, 14.00000000000000000 ) ) ;
#2468=CARTESIAN_POINT ( 'NONE',  ( -9.247353065533557626, -2.155497948345702408, 1.999999999999998224 ) ) ;
#2471=CARTESIAN_POINT ( 'NONE',  ( -6.667513054348624735, -4.302816426345351886, 1.999999999999998224 ) ) ;
#2474=CARTESIAN_POINT ( 'NONE',  ( 5.887534416617372202, 3.663839002572494952, 13.99999999999999645 ) ) ;
#2475=B_SPLINE_CURVE_WITH_KNOTS ( 'NONE', 3,
 ( #1377, #1746, #3133, #2233, #3905, #3517, #883, #1292, #4881, #423, #3501, #365, #4855, #3988, #3023, #5262, #1316, #3937, #854, #3077, #4822, #48, #2670, #2642, #4339, #1722, #3475, #938, #4396, #4421, #1773, #20, #2181, #2122, #451, #1687, #2210, #1803, #3559, #3444, #1261, #4315, #390, #5236, #3050, #3876, #3528, #4793, #4767, #3961, #2150, #5290, #5318, #1347, #828, #5202, #2580, #5661, #3106, #911, #4369, #969, #3750, #265, #1590, #997, #2024, #1832, #1401, #705, #4641, #3590, #4155, #5343, #1430, #2395, #3716, #506, #4049, #2263, #2885, #1962, #3294, #3350, #2727, #5507, #3778, #5103, #2756, #5534, #3163, #4909, #2457, #4215, #4478, #209, #538, #3189, #5476, #1537, #4020, #2859, #2423, #4185, #2692, #4448, #4940, #5042, #2289, #644, #77, #103, #1860, #3616, #5373, #4586, #1102, #4612, #671, #237, #1997, #1566, #3322, #5069, #1128, #3406, #5645, #839, #351, #4352, #4268, #4694, #1161, #2048, #2972, #3921, #406, #2165, #5134, #4779, #5615, #755, #4669, #730, #320, #3863, #3034, #2080, #1244, #3805, #3430, #2536, #4720, #2942, #3486, #4299, #5591, #4751, #2916, #5674, #3838, #5562, #2106, #1675, #783, #5158, #5185, #3005, #814, #1735, #2566, #4326, #1650, #2506, #2483, #1218, #375, #2136, #3890, #1704, #1621, #3458, #4239, #5222, #2594, #290, #3381, #1192, #1279, #4922, #5303, #4838, #1389, #5248, #2743, #2275, #1845, #115, #4063, #4004, #3601, #2194, #868, #4494, #3948, #61, #1819, #2710, #4462, #439, #89, #4035, #1364, #4804, #3120, #2221, #32, #2627, #1871, #1329, #462, #3146, #1304, #548, #5355, #1412, #3062, #4382, #3575, #3175, #487, #1786, #3092, #898, #983, #2302, #2655, #7, #3543, #3972, #1757, #3513 ),
 .UNSPECIFIED., .F., .F.,
 ( 4, 2, 2, 2, 2, 2, 2, 2, 2, 2, 2, 2, 2, 2, 2, 2, 2, 2, 2, 2, 2, 2, 2, 2, 2, 2, 2, 2, 2, 2, 2, 2, 2, 2, 2, 2, 2, 2, 2, 2, 2, 2, 2, 2, 2, 2, 2, 2, 2, 2, 2, 2, 2, 2, 2, 2, 2, 2, 2, 2, 2, 2, 2, 2, 2, 2, 2, 2, 2, 2, 2, 2, 2, 2, 2, 2, 2, 2, 2, 2, 2, 2, 2, 2, 2, 2, 2, 2, 2, 2, 2, 2, 2, 2, 2, 2, 2, 2, 2, 2, 2, 2, 2, 2, 2, 2, 2, 2, 2, 2, 2, 2, 2, 2, 2, 2, 2, 2, 2, 2, 4 ),
 ( 0.000000000000000000, 0.01562500000000000000, 0.03125000000000000000, 0.04687500000000000000, 0.06250000000000000000, 0.07812500000000000000, 0.09375000000000000000, 0.1093750000000000000, 0.1250000000000000000, 0.1328125000000000000, 0.1406250000000000000, 0.1484375000000000000, 0.1562500000000000000, 0.1640625000000000000, 0.1718750000000000000, 0.1796875000000000000, 0.1875000000000000000, 0.1953125000000000000, 0.2031250000000000000, 0.2109375000000000000, 0.2187500000000000000, 0.2265625000000000000, 0.2343750000000000000, 0.2421875000000000000, 0.2500000000000000000, 0.2578125000000000000, 0.2656250000000000000, 0.2734375000000000000, 0.2812500000000000000, 0.2890625000000000000, 0.2968750000000000000, 0.3046875000000000000, 0.3125000000000000000, 0.3203125000000000000, 0.3281250000000000000, 0.3359375000000000000, 0.3437500000000000000, 0.3515625000000000000, 0.3593750000000000000, 0.3671875000000000000, 0.3750000000000000000, 0.3828125000000000000, 0.3906250000000000000, 0.3984375000000000000, 0.4062500000000000000, 0.4140625000000000000, 0.4218750000000000000, 0.4296875000000000000, 0.4375000000000000000, 0.4453125000000000000, 0.4531250000000000000, 0.4609375000000000000, 0.4687500000000000000, 0.4765625000000000000, 0.4843750000000000000, 0.4921875000000000000, 0.5000000000000000000, 0.5078125000000000000, 0.5156250000000000000, 0.5234375000000000000, 0.5312500000000000000, 0.5390625000000000000, 0.5468750000000000000, 0.5546875000000000000, 0.5625000000000000000, 0.5703125000000000000, 0.5781250000000000000, 0.5859375000000000000, 0.5937500000000000000, 0.6015625000000000000, 0.6093750000000000000, 0.6171875000000000000, 0.6250000000000000000, 0.6328125000000000000, 0.6406250000000000000, 0.6484375000000000000, 0.6562500000000000000, 0.6640625000000000000, 0.6718750000000000000, 0.6796875000000000000, 0.6875000000000000000, 0.6953125000000000000, 0.7031250000000000000, 0.7109375000000000000, 0.7187500000000000000, 0.7265625000000000000, 0.7343750000000000000, 0.7421875000000000000, 0.7500000000000000000, 0.7578125000000000000, 0.7656250000000000000, 0.7734375000000000000, 0.7812500000000000000, 0.7890625000000000000, 0.7968750000000000000, 0.8046875000000000000, 0.8125000000000000000, 0.8203125000000000000, 0.8281250000000000000, 0.8359375000000000000, 0.8437500000000000000, 0.8515625000000000000, 0.8593750000000000000, 0.8671875000000000000, 0.8750000000000000000, 0.8828125000000000000, 0.8906250000000000000, 0.8984375000000000000, 0.9062500000000000000, 0.9140625000000000000, 0.9218750000000000000, 0.9296875000000000000, 0.9375000000000000000, 0.9453125000000000000, 0.9531250000000000000, 0.9609375000000000000, 0.9687500000000000000, 0.9765625000000000000, 0.9843750000000000000, 0.9921875000000000000, 1.000000000000000000 ),
 .UNSPECIFIED. ) ;
#2482=CARTESIAN_POINT ( 'NONE',  ( -8.745075223330342595, 3.959260399367897421, 1.999999999999998224 ) ) ;
#2483=CARTESIAN_POINT ( 'NONE',  ( -3.127066335681350395, 9.214240776398044730, 13.99999999999999645 ) ) ;
#2484=CARTESIAN_POINT ( 'NONE',  ( -8.332455577112462208, 5.761155596212925722, 14.00000000000000000 ) ) ;
#2485=EDGE_CURVE ( 'NONE', #261, #660, #4914, .T. ) ;
#2490=CARTESIAN_POINT ( 'NONE',  ( 3.520917041835319505, -6.848083076131263880, 14.00000000000000000 ) ) ;
#2491=CARTESIAN_POINT ( 'NONE',  ( 1.954797901281673633, -9.037865403626287986, 13.99999999999999645 ) ) ;
#2492=CARTESIAN_POINT ( 'NONE',  ( -4.089163901200158158, 5.898691170884823975, 14.00000000000000000 ) ) ;
#2494=CARTESIAN_POINT ( 'NONE',  ( 7.233280636258586860, 6.778630567624379211, 1.999999999999998224 ) ) ;
#2495=CARTESIAN_POINT ( 'NONE',  ( 2.369394374793902802, -7.353877281245869035, 1.999999999999998224 ) ) ;
#2497=CARTESIAN_POINT ( 'NONE',  ( -2.919577271296576182, -6.733962781534541975, 13.99999999999999645 ) ) ;
#2498=( GEOMETRIC_REPRESENTATION_CONTEXT ( 3 ) GLOBAL_UNCERTAINTY_ASSIGNED_CONTEXT ( ( #3112 ) ) GLOBAL_UNIT_ASSIGNED_CONTEXT ( ( #3372, #3829, #3140 ) ) REPRESENTATION_CONTEXT ( 'NONE', 'WORKASPACE' ) );
#2499=CARTESIAN_POINT ( 'NONE',  ( 9.522148329495122354, -0.6196525284525815636, 1.999999999999998224 ) ) ;
#2506=CARTESIAN_POINT ( 'NONE',  ( -3.867583043141954224, 8.914321633329153727, 13.99999999999999645 ) ) ;
#2507=CARTESIAN_POINT ( 'NONE',  ( -7.304208470128496167, 7.056621303512280896, 14.00000000000000000 ) ) ;
#2512=CARTESIAN_POINT ( 'NONE',  ( -3.715337444063475658, -5.771435016728993617, 14.00000000000000000 ) ) ;
#2513=CARTESIAN_POINT ( 'NONE',  ( -10.42442484909544653, -1.371544430045602558, 13.99999999999999645 ) ) ;
#2515=CARTESIAN_POINT ( 'NONE',  ( 5.195030181282107584, -4.117271336869512410, 14.00000000000000000 ) ) ;
#2518=CARTESIAN_POINT ( 'NONE',  ( -7.080399483669990168, -6.208478756603781790, 1.999999999999998224 ) ) ;
#2521=CARTESIAN_POINT ( 'NONE',  ( 4.415008247871750058, 7.106745273741266189, 1.999999999999998224 ) ) ;
#2525=CARTESIAN_POINT ( 'NONE',  ( 5.806279480217827249, -1.975834710110474512, 1.999999999999998224 ) ) ;
#2526=CARTESIAN_POINT ( 'NONE',  ( 2.406079317367887604, 6.392288322179703108, 13.99999999999999645 ) ) ;
#2528=CARTESIAN_POINT ( 'NONE',  ( 5.519166806814063797, -7.959527472085689226, 1.999999999999998224 ) ) ;
#2536=CARTESIAN_POINT ( 'NONE',  ( -0.3010823416051303103, -9.281161307073869438, 13.99999999999999645 ) ) ;
#2543=CARTESIAN_POINT ( 'NONE',  ( 7.925371078819432036, 2.990572132494779378, 14.00000000000000000 ) ) ;
#2545=CARTESIAN_POINT ( 'NONE',  ( 4.914575889516862972, -3.754581871930560144, 1.999999999999998224 ) ) ;
#2549=CARTESIAN_POINT ( 'NONE',  ( -7.019001384594682591, 0.4577903460187995877, 14.00000000000000000 ) ) ;
#2552=CARTESIAN_POINT ( 'NONE',  ( -5.337360893037004672, -7.710592058383595848, 1.999999999999998224 ) ) ;
#2556=CARTESIAN_POINT ( 'NONE',  ( 7.320916985966518631, 1.587212364775676843, 1.999999999999998224 ) ) ;
#2558=CARTESIAN_POINT ( 'NONE',  ( -4.310533329768688304, 5.077046166951620698, 1.999999999999412914 ) ) ;
#2559=CARTESIAN_POINT ( 'NONE',  ( -5.978927507574435474, 2.933119789328458182, 13.99999999999999645 ) ) ;
#2560=CARTESIAN_POINT ( 'NONE',  ( 0.1634456542307745064, 10.28566380800474533, 1.999999999999998224 ) ) ;
#2566=CARTESIAN_POINT ( 'NONE',  ( -7.044187934146358465, 6.598551529630926282, 13.99999999999999645 ) ) ;
#2571=ORIENTED_EDGE ( 'NONE', *, *, #3073, .F. ) ;
#2573=CARTESIAN_POINT ( 'NONE',  ( -6.826495404309340209, 4.393449859560456083, 14.00000000000000000 ) ) ;
#2574=CARTESIAN_POINT ( 'NONE',  ( -7.035243215357270152, 8.023489478516461659, 13.99999999999999645 ) ) ;
#2575=PRODUCT_DEFINITION_CONTEXT ( 'detailed design', #2102, 'design' ) ;
#2576=DIRECTION ( 'NONE',  ( -0.000000000000000000, 1.000000000000000000, 0.000000000000000000 ) ) ;
#2577=CARTESIAN_POINT ( 'NONE',  ( -6.826495404309340209, 4.393449859560456083, 14.00000000000000000 ) ) ;
#2579=CARTESIAN_POINT ( 'NONE',  ( 7.456063200420987691, 7.959410280423138140, 1.999999999999998224 ) ) ;
#2580=CARTESIAN_POINT ( 'NONE',  ( -5.810612947750823487, -4.611264106266947493, 13.99999999999999645 ) ) ;
#2582=CARTESIAN_POINT ( 'NONE',  ( -6.185289998984973003, -6.402116997106289453, 1.999999999999998224 ) ) ;
#2583=CARTESIAN_POINT ( 'NONE',  ( -0.5931392160223127874, -7.263020831007572120, 1.999999999999998224 ) ) ;
#2584=CARTESIAN_POINT ( 'NONE',  ( 8.164254108709979363, -4.026826083952141921, 13.99999999999999645 ) ) ;
#2585=MANIFOLD_SOLID_BREP ( 'Sweep1', #510 ) ;
#2587=CARTESIAN_POINT ( 'NONE',  ( 1.124407659250306279, -9.699258357302506184, 1.999999999999998224 ) ) ;
#2594=CARTESIAN_POINT ( 'NONE',  ( 7.775655769254120386, 6.170250810330326630, 13.99999999999999645 ) ) ;
#2601=CARTESIAN_POINT ( 'NONE',  ( -5.581220830679986200, 5.949058968288507110, 14.00000000000000000 ) ) ;
#2602=CARTESIAN_POINT ( 'NONE',  ( -1.424809953814531127, 6.586142414399820844, 1.999999999999998224 ) ) ;
#2605=CARTESIAN_POINT ( 'NONE',  ( 3.810368753942760200, 7.433568398487740758, 14.00000000000000000 ) ) ;
#2611=SHAPE_DEFINITION_REPRESENTATION ( #269, #4116 ) ;
#2612=CARTESIAN_POINT ( 'NONE',  ( 9.527640065893086430, 0.1642265212908741445, 1.999999999999998224 ) ) ;
#2613=CARTESIAN_POINT ( 'NONE',  ( 7.409328306158467825, 2.927536720054290775, 1.999999999999998224 ) ) ;
#2614=CARTESIAN_POINT ( 'NONE',  ( 7.132151089625189400, 3.519983721611798622, 13.99999999999999645 ) ) ;
#2623=CARTESIAN_POINT ( 'NONE',  ( 3.896371052708264227, -4.167854722424304548, 1.999999999999998224 ) ) ;
#2626=MECHANICAL_DESIGN_GEOMETRIC_PRESENTATION_REPRESENTATION('',(#1053),#47);
#2627=CARTESIAN_POINT ( 'NONE',  ( -10.17357856257779680, 2.902115915870757679, 13.99999999999999645 ) ) ;
#2634=CARTESIAN_POINT ( 'NONE',  ( -7.963215149404076598, -4.094909132697305054, 14.00000000000000000 ) ) ;
#2635=CARTESIAN_POINT ( 'NONE',  ( -0.4015567206217142693, -6.330257989742454683, 1.999999999999998224 ) ) ;
#2638=CARTESIAN_POINT ( 'NONE',  ( -2.020383375745357313, -7.552201994671271734, 14.00000000000000000 ) ) ;
#2640=AXIS2_PLACEMENT_3D ( 'NONE', #3946, #2274, #1784 ) ;
#2641=CARTESIAN_POINT ( 'NONE',  ( 5.279590631141700463, 9.498297537454860162, 1.999999999999998224 ) ) ;
#2642=CARTESIAN_POINT ( 'NONE',  ( 0.2194671214740386012, 6.774136816532214667, 13.99999999999999645 ) ) ;
#2645=CARTESIAN_POINT ( 'NONE',  ( 8.370269057507494281, -1.803949267857694716, 1.999999999999998224 ) ) ;
#2647=CARTESIAN_POINT ( 'NONE',  ( -2.122668041763332347, 7.434468402752582250, 1.999999999999998224 ) ) ;
#2655=CARTESIAN_POINT ( 'NONE',  ( 9.199536834907137361, 5.930433524308741156, 13.99999999999999645 ) ) ;
#2657=CARTESIAN_POINT ( 'NONE',  ( 6.000000000000001776, 0.000000000000000000, 13.99999999999999645 ) ) ;
#2658=ORIENTED_EDGE ( 'NONE', *, *, #1888, .T. ) ;
#2660=CARTESIAN_POINT ( 'NONE',  ( 7.311638624438943523, 4.225618826270838291, 14.00000000000000000 ) ) ;
#2661=CARTESIAN_POINT ( 'NONE',  ( 1.015216742983932274, 7.730330528320553896, 1.999999999999998224 ) ) ;
#2665=CARTESIAN_POINT ( 'NONE',  ( 1.147089839255721166, -8.682979827542890661, 14.00000000000000000 ) ) ;
#2667=CARTESIAN_POINT ( 'NONE',  ( 10.02239396097947655, -0.6576683464576721372, 1.999999999999998224 ) ) ;
#2668=CARTESIAN_POINT ( 'NONE',  ( 0.1774200004017884857, 10.78715707688374614, 1.999999999999998224 ) ) ;
#2670=CARTESIAN_POINT ( 'NONE',  ( -0.8811140424828162176, 6.693995663234412419, 13.99999999999999645 ) ) ;
#2671=CARTESIAN_POINT ( 'NONE',  ( 5.519166806814063797, -7.959527472085689226, 1.999999999999998224 ) ) ;
#2672=CARTESIAN_POINT ( 'NONE',  ( 3.909482108038854431, 5.648312977191785045, 1.999999999999998224 ) ) ;
#2676=CARTESIAN_POINT ( 'NONE',  ( 4.815977876496239318, 4.225366587634176163, 1.999999999999998224 ) ) ;
#2684=CARTESIAN_POINT ( 'NONE',  ( -8.290222237439158093, 3.747600907060152586, 14.00000000000000000 ) ) ;
#2685=CARTESIAN_POINT ( 'NONE',  ( 8.027649061863494140, -0.2602747315786821392, 1.999999999999998224 ) ) ;
#2686=CARTESIAN_POINT ( 'NONE',  ( 8.518575158373787204, 0.2826087140540892162, 1.999999999999998224 ) ) ;
#2687=CARTESIAN_POINT ( 'NONE',  ( -7.301858691287087311, -3.172613069824385956, 14.00000000000000000 ) ) ;
#2689=CARTESIAN_POINT ( 'NONE',  ( -5.893815055328603947, 7.676334994785346311, 1.999999999999998224 ) ) ;
#2690=CARTESIAN_POINT ( 'NONE',  ( 10.98697916625148707, 0.8999353979983775176, 1.999999999999998224 ) ) ;
#2692=CARTESIAN_POINT ( 'NONE',  ( -4.060726170632903198, -7.305992298388080286, 13.99999999999999645 ) ) ;
#2694=CARTESIAN_POINT ( 'NONE',  ( 1.853537052132013363, -8.546502713975391075, 1.999999999999998224 ) ) ;
#2696=CARTESIAN_POINT ( 'NONE',  ( 1.649120185255090298, 7.633850905136056575, 1.999999999999998224 ) ) ;
#2701=( NAMED_UNIT ( * ) SI_UNIT ( $, .STERADIAN. ) SOLID_ANGLE_UNIT ( ) );
#2703=CARTESIAN_POINT ( 'NONE',  ( 4.513069810084762601, -3.445129632735342451, 1.999999999999998224 ) ) ;
#2710=CARTESIAN_POINT ( 'NONE',  ( -6.045729098460493667, -8.441868823237593134, 13.99999999999999645 ) ) ;
#2716=CARTESIAN_POINT ( 'NONE',  ( -9.986481889892992569, 1.144076113142371787, 14.00000000000000000 ) ) ;
#2717=CARTESIAN_POINT ( 'NONE',  ( 6.638644669766898154, 2.135480210976827387, 1.999999999999998224 ) ) ;
#2719=CARTESIAN_POINT ( 'NONE',  ( 0.5385325299235221852, 8.270587056550796845, 1.999999999999998224 ) ) ;
#2720=CARTESIAN_POINT ( 'NONE',  ( 9.164356920906893578, 2.464151434935829332, 14.00000000000000000 ) ) ;
#2723=CARTESIAN_POINT ( 'NONE',  ( -5.651290410005069376, 9.082320918485367045, 1.999999999999998224 ) ) ;
#2724=CARTESIAN_POINT ( 'NONE',  ( 6.315449825284095375, 1.474116854620425299, 14.00000000000000000 ) ) ;
#2725=CARTESIAN_POINT ( 'NONE',  ( -8.440272934376814362, 1.393994921405934173, 13.99999999999999645 ) ) ;
#2727=CARTESIAN_POINT ( 'NONE',  ( 7.409328306158469601, 2.927536720054149555, 13.99999999999999645 ) ) ;
#2728=CARTESIAN_POINT ( 'NONE',  ( -1.336592501075063666, -5.709464570123372162, 14.00000000000000000 ) ) ;
#2731=CARTESIAN_POINT ( 'NONE',  ( 5.381714297850622053, -6.137309488907494170, 1.999999999999998224 ) ) ;
#2740=CARTESIAN_POINT ( 'NONE',  ( -6.069783318623453106, -0.2142533344232669390, 1.999999999999998224 ) ) ;
#2743=CARTESIAN_POINT ( 'NONE',  ( 8.595497693524210447, -5.345940745659388149, 13.99999999999999645 ) ) ;
#2748=CARTESIAN_POINT ( 'NONE',  ( 9.522148329495834673, -0.6196525284526704924, 14.00000000000000000 ) ) ;
#2749=CARTESIAN_POINT ( 'NONE',  ( -5.745624475482103755, 5.035517847229626476, 1.999999999999998224 ) ) ;
#2750=CARTESIAN_POINT ( 'NONE',  ( -8.547479018124427341, -2.754496926847987748, 1.999999999999998224 ) ) ;
#2751=CARTESIAN_POINT ( 'NONE',  ( 1.124407659250215685, -9.699258357303232714, 14.00000000000000000 ) ) ;
#2753=CARTESIAN_POINT ( 'NONE',  ( -7.660583958272733973, 7.409732212660907535, 1.999999999999998224 ) ) ;
#2755=CARTESIAN_POINT ( 'NONE',  ( 8.859712399101631775, -1.914114158827161294, 13.99999999999999645 ) ) ;
#2756=CARTESIAN_POINT ( 'NONE',  ( 7.992346231215207375, -0.9198489573344114101, 13.99999999999999645 ) ) ;
#2757=CARTESIAN_POINT ( 'NONE',  ( -8.072272399572318236, -5.790267008923112080, 1.999999999999998224 ) ) ;
#2759=CARTESIAN_POINT ( 'NONE',  ( 8.952336951391263398, 1.032601321559316832, 1.999999999999998224 ) ) ;
#2760=( NAMED_UNIT ( * ) PLANE_ANGLE_UNIT ( ) SI_UNIT ( $, .RADIAN. ) );
#2763=CARTESIAN_POINT ( 'NONE',  ( 5.195030181282357162, -4.117271336869386289, 1.999999999999998224 ) ) ;
#2765=CARTESIAN_POINT ( 'NONE',  ( -6.876639332705558161, 1.598006320995754237, 1.999999999999998224 ) ) ;
#2768=APPLICATION_CONTEXT ( 'automotive_design' ) ;
#2772=CARTESIAN_POINT ( 'NONE',  ( 7.379526280503350577, 5.862399640741291940, 14.00000000000000000 ) ) ;
#2773=CARTESIAN_POINT ( 'NONE',  ( -6.792624376349762905, -3.077375260546124203, 1.999999999999998224 ) ) ;
#2774=CARTESIAN_POINT ( 'NONE',  ( -4.424777426321968576, -7.679192617323552739, 1.999999999999998224 ) ) ;
#2775=CARTESIAN_POINT ( 'NONE',  ( -9.926332099419621358, -1.311590842189569894, 14.00000000000000000 ) ) ;
#2777=CARTESIAN_POINT ( 'NONE',  ( -1.592064345877699072, 9.625584969238365929, 1.999999999999998224 ) ) ;
#2778=CARTESIAN_POINT ( 'NONE',  ( -3.922355934210178585, -4.464780306277046584, 14.00000000000000000 ) ) ;
#2779=CARTESIAN_POINT ( 'NONE',  ( -6.848710654519975627, 5.255840572796830479, 13.99999999999999645 ) ) ;
#2781=CARTESIAN_POINT ( 'NONE',  ( 0.2014543481397604030, 6.272771216426900942, 14.00000000000000000 ) ) ;
#2783=CARTESIAN_POINT ( 'NONE',  ( -4.227552200850895225, 7.601683304540809871, 1.999999999999998224 ) ) ;
#2785=CARTESIAN_POINT ( 'NONE',  ( 0.2014543481397604585, 6.272771216426899166, 1.999999999999998224 ) ) ;
#2787=CARTESIAN_POINT ( 'NONE',  ( -7.019001384594680815, 0.4577903460188660345, 1.999999999999998224 ) ) ;
#2800=CARTESIAN_POINT ( 'NONE',  ( -8.929154442179243034, -4.413097966322579779, 14.00000000000000000 ) ) ;
#2801=CARTESIAN_POINT ( 'NONE',  ( 5.381714297850622053, -6.137309488907494170, 1.999999999999998224 ) ) ;
#2802=CARTESIAN_POINT ( 'NONE',  ( -4.895455514773497718, -6.178604150901914061, 1.999999999999998224 ) ) ;
#2803=CARTESIAN_POINT ( 'NONE',  ( -1.271096247112511346, -9.720655361064800104, 14.00000000000000000 ) ) ;
#2809=CARTESIAN_POINT ( 'NONE',  ( 4.443413384189735638, 4.597174039215665253, 14.00000000000000000 ) ) ;
#2810=CARTESIAN_POINT ( 'NONE',  ( 1.176163838800443395, -10.19826953922044765, 13.99999999999999645 ) ) ;
#2811=CARTESIAN_POINT ( 'NONE',  ( -5.021280548128706833, 3.603657539914777885, 14.00000000000094147 ) ) ;
#2814=CARTESIAN_POINT ( 'NONE',  ( -5.741039858921414663, -6.128965587877393872, 1.999999999999998224 ) ) ;
#2819=CARTESIAN_POINT ( 'NONE',  ( 6.445330636073144603, -1.168293168414208827, 1.999999999999998224 ) ) ;
#2821=CARTESIAN_POINT ( 'NONE',  ( 5.499810765991186123, -5.314180015047517358, 1.999999999999998224 ) ) ;
#2824=CARTESIAN_POINT ( 'NONE',  ( 4.243312049792015372, -4.537448458213933833, 13.99999999999999645 ) ) ;
#2833=CARTESIAN_POINT ( 'NONE',  ( 8.859712399100347469, -1.914114158827000312, 1.999999999999998224 ) ) ;
#2835=CARTESIAN_POINT ( 'NONE',  ( 3.713512749562912774, 8.576920285552665391, 1.999999999999998224 ) ) ;
#2836=CARTESIAN_POINT ( 'NONE',  ( -4.424777426322135554, -7.679192617324877901, 14.00000000000000000 ) ) ;
#2839=CARTESIAN_POINT ( 'NONE',  ( 10.06493078320224832, 4.366638945733749111, 1.999999999999998224 ) ) ;
#2840=CARTESIAN_POINT ( 'NONE',  ( -6.048456868091351524, 0.8014113234714785872, 14.00000000000000000 ) ) ;
#2841=CARTESIAN_POINT ( 'NONE',  ( 4.074896204546096357, -8.256886768010264888, 13.99999999999999645 ) ) ;
#2843=CARTESIAN_POINT ( 'NONE',  ( -8.765969750979122566, 5.050798838973363125, 1.999999999999998224 ) ) ;
#2845=CARTESIAN_POINT ( 'NONE',  ( -6.848710654519973851, 5.255840572796829591, 1.999999999999998224 ) ) ;
#2848=CARTESIAN_POINT ( 'NONE',  ( -3.987231204391976203, 4.693390172671164429, 1.999999999999412914 ) ) ;
#2850=CARTESIAN_POINT ( 'NONE',  ( 3.247347166530788698, 6.590896817052186663, 1.999999999999998224 ) ) ;
#2852=CARTESIAN_POINT ( 'NONE',  ( -0.4015567206216588692, -6.330257989742014146, 13.99999999999999645 ) ) ;
#2857=CARTESIAN_POINT ( 'NONE',  ( 9.602236826902712963, 4.172718697305597857, 14.00000000000000000 ) ) ;
#2858=CARTESIAN_POINT ( 'NONE',  ( 6.971023843911450690, -5.915260676233723203, 1.999999999999998224 ) ) ;
#2859=CARTESIAN_POINT ( 'NONE',  ( -1.484422800923361985, -8.172499773498691056, 13.99999999999999645 ) ) ;
#2860=CARTESIAN_POINT ( 'NONE',  ( 4.264126983937992499, 9.433107915010287670, 14.00000000000000000 ) ) ;
#2865=CARTESIAN_POINT ( 'NONE',  ( 7.494325059173605474, -0.8592991332473474131, 14.00000000000000000 ) ) ;
#2867=CARTESIAN_POINT ( 'NONE',  ( -4.679820741050984445, -8.111215689329295486, 13.99999999999999645 ) ) ;
#2868=CARTESIAN_POINT ( 'NONE',  ( -1.105557477332586691, -6.708264047591377732, 14.00000000000000000 ) ) ;
#2869=VERTEX_POINT ( 'NONE', #5047 ) ;
#2870=CARTESIAN_POINT ( 'NONE',  ( -10.26372689808571970, -2.219791875069699216, 1.999999999999998224 ) ) ;
#2873=CARTESIAN_POINT ( 'NONE',  ( 3.622712361020122618, 5.236663886535374957, 1.999999999999998224 ) ) ;
#2875=CARTESIAN_POINT ( 'NONE',  ( 0.5542950790998156796, -6.736796398737814329, 1.999999999999998224 ) ) ;
#2876=CARTESIAN_POINT ( 'NONE',  ( -4.256527737015712631, -4.845957569453684499, 1.999999999999998224 ) ) ;
#2883=CARTESIAN_POINT ( 'NONE',  ( -3.290073422422500560, -8.739709727800574868, 1.999999999999998224 ) ) ;
#2885=CARTESIAN_POINT ( 'NONE',  ( 5.103689747953259470, 6.014827819656690444, 13.99999999999999645 ) ) ;
#2891=CARTESIAN_POINT ( 'NONE',  ( 8.671201137383034663, 6.657490096169006222, 1.999999999999998224 ) ) ;
#2893=CARTESIAN_POINT ( 'NONE',  ( 0.9466184546083361573, 7.233353930637703044, 14.00000000000000000 ) ) ;
#2894=CARTESIAN_POINT ( 'NONE',  ( 6.971023843911450690, -5.915260676233724091, 13.99999999999999645 ) ) ;
#2895=VECTOR ( 'NONE', #1003, 1000.000000000000000 ) ;
#2897=CARTESIAN_POINT ( 'NONE',  ( 6.340368144647111848, -1.697206311171021831, 14.00000000000000000 ) ) ;
#2899=CARTESIAN_POINT ( 'NONE',  ( 3.917689075872947235, 9.035181080458078995, 1.999999999999998224 ) ) ;
#2903=CARTESIAN_POINT ( 'NONE',  ( -3.391372024942433505, 7.476497417048837413, 1.999999999999998224 ) ) ;
#2905=CARTESIAN_POINT ( 'NONE',  ( 0.5141566911143078400, -7.748312628312726602, 1.999999999999998224 ) ) ;
#2906=CARTESIAN_POINT ( 'NONE',  ( 0.7762864403411611214, 6.746413643992394960, 1.999999999999998224 ) ) ;
#2907=CARTESIAN_POINT ( 'NONE',  ( -0.2539011084976132149, 7.766605221862832309, 13.99999999999999645 ) ) ;
#2908=EDGE_CURVE ( 'NONE', #660, #2869, #1105, .T. ) ;
#2909=DIRECTION ( 'NONE',  ( 0.9999273757268464236, -0.01205169166640781934, 0.000000000000000000 ) ) ;
#2914=CARTESIAN_POINT ( 'NONE',  ( -3.594774944545354511, 7.935102286573618713, 1.999999999999998224 ) ) ;
#2916=CARTESIAN_POINT ( 'NONE',  ( -7.080399483669658878, -6.208478756603783566, 13.99999999999999645 ) ) ;
#2923=CARTESIAN_POINT ( 'NONE',  ( -6.881333183081246752, -1.254343363641206688, 14.00000000000000000 ) ) ;
#2924=CARTESIAN_POINT ( 'NONE',  ( 7.233280636258937690, 6.778630567624380099, 13.99999999999999645 ) ) ;
#2925=CARTESIAN_POINT ( 'NONE',  ( -4.975175822334874098, 5.137265612443751017, 14.00000000000000000 ) ) ;
#2927=CARTESIAN_POINT ( 'NONE',  ( 9.077580196902394150, 4.112174628513753483, 1.999999999999998224 ) ) ;
#2931=CARTESIAN_POINT ( 'NONE',  ( 7.494325059173603698, -0.8592991332473469690, 1.999999999999998224 ) ) ;
#2933=CARTESIAN_POINT ( 'NONE',  ( 6.180183843827204093, 3.174252413088802793, 13.99999999999999645 ) ) ;
#2935=CARTESIAN_POINT ( 'NONE',  ( -3.609299841826103972, -9.156952235374472338, 1.999999999999998224 ) ) ;
#2941=CARTESIAN_POINT ( 'NONE',  ( -9.247353065533557626, -2.155497948345702408, 1.999999999999998224 ) ) ;
#2942=CARTESIAN_POINT ( 'NONE',  ( -2.557952627993306471, -8.967547948949398773, 13.99999999999999645 ) ) ;
#2948=CARTESIAN_POINT ( 'NONE',  ( 2.690160903457257557, 6.823041841979409661, 14.00000000000000000 ) ) ;
#2949=CARTESIAN_POINT ( 'NONE',  ( 6.769338797470518365, 8.534199679355843671, 13.99999999999999645 ) ) ;
#2951=CARTESIAN_POINT ( 'NONE',  ( 7.494325059173605474, -0.8592991332473474131, 14.00000000000000000 ) ) ;
#2954=CARTESIAN_POINT ( 'NONE',  ( 0.3355163285737912116, -10.27362971114624024, 1.999999999999998224 ) ) ;
#2959=CARTESIAN_POINT ( 'NONE',  ( -7.425829140954076202, 3.215541426300492223, 1.999999999999998224 ) ) ;
#2961=CARTESIAN_POINT ( 'NONE',  ( -0.5931392160223127874, -7.263020831007573896, 13.99999999999999645 ) ) ;
#2964=CARTESIAN_POINT ( 'NONE',  ( 6.721134410589269415, -6.938257756003234356, 1.999999999999998224 ) ) ;
#2972=CARTESIAN_POINT ( 'NONE',  ( 7.748217264258252968, 4.472783157626409434, 13.99999999999999645 ) ) ;
#2973=CARTESIAN_POINT ( 'NONE',  ( -8.765969750978372943, 5.050798838973364902, 14.00000000000000000 ) ) ;
#2978=CARTESIAN_POINT ( 'NONE',  ( 3.810368753942760200, 7.433568398487740758, 14.00000000000000000 ) ) ;
#2979=CARTESIAN_POINT ( 'NONE',  ( -3.886954398759499885, 5.424498719065524277, 1.999999999999998224 ) ) ;
#2983=CARTESIAN_POINT ( 'NONE',  ( 4.776808680784973227, 5.634249062854204126, 14.00000000000000000 ) ) ;
#2986=CARTESIAN_POINT ( 'NONE',  ( -9.381622446299669349, -4.629808687489259889, 1.999999999999998224 ) ) ;
#2991=CARTESIAN_POINT ( 'NONE',  ( 8.453438707198472457, 0.9797652757261496870, 1.999999999999998224 ) ) ;
#2994=CARTESIAN_POINT ( 'NONE',  ( -1.424809953814591523, 6.586142414399822620, 13.99999999999999645 ) ) ;
#2997=DIRECTION ( 'NONE',  ( 0.000000000000000000, 0.000000000000000000, 1.000000000000000000 ) ) ;
#2998=CARTESIAN_POINT ( 'NONE',  ( -0.7616497023963333390, 9.236585841460744462, 1.999999999999998224 ) ) ;
#3005=CARTESIAN_POINT ( 'NONE',  ( -8.745075223331019387, 3.959260399367729111, 13.99999999999999645 ) ) ;
#3009=CARTESIAN_POINT ( 'NONE',  ( 10.50003631213657940, 0.006025845833179013789, 7.999999999999998224 ) ) ;
#3013=CARTESIAN_POINT ( 'NONE',  ( -7.301858691287087311, -3.172613069824385956, 14.00000000000000000 ) ) ;
#3015=CARTESIAN_POINT ( 'NONE',  ( -1.451466707715830973, -6.203196315423896934, 1.999999999999998224 ) ) ;
#3018=CARTESIAN_POINT ( 'NONE',  ( 5.499810765991187012, -5.314180015047230476, 14.00000000000000000 ) ) ;
#3020=CARTESIAN_POINT ( 'NONE',  ( -3.287100391418392942, 10.22059872437900019, 1.999999999999998224 ) ) ;
#3023=CARTESIAN_POINT ( 'NONE',  ( -6.551010013419181988, 0.8677952034721571062, 13.99999999999999645 ) ) ;
#3025=CARTESIAN_POINT ( 'NONE',  ( -8.013356705133178437, 0.6503825268544296545, 1.999999999999998224 ) ) ;
#3026=CARTESIAN_POINT ( 'NONE',  ( 6.209839678910233474, -3.451293940533043614, 1.999999999999998224 ) ) ;
#3027=CARTESIAN_POINT ( 'NONE',  ( -7.519441789400338472, 0.4931591957933217363, 13.99999999999999645 ) ) ;
#3029=CARTESIAN_POINT ( 'NONE',  ( -6.681386044268610824, 6.252046474378027519, 1.999999999999998224 ) ) ;
#3034=CARTESIAN_POINT ( 'NONE',  ( 5.347643153870340171, -7.463670412150953837, 13.99999999999999645 ) ) ;
#3040=CARTESIAN_POINT ( 'NONE',  ( -1.001529162299639619, -8.740421795711004194, 14.00000000000000000 ) ) ;
#3041=CARTESIAN_POINT ( 'NONE',  ( -8.741731599017841248, 6.051300285686072478, 13.99999999999999645 ) ) ;
#3044=CARTESIAN_POINT ( 'NONE',  ( -3.813875884798381577, -6.869235835554827752, 14.00000000000000000 ) ) ;
#3050=CARTESIAN_POINT ( 'NONE',  ( 3.892125705850195683, -6.036954802193643665, 13.99999999999999645 ) ) ;
#3051=CARTESIAN_POINT ( 'NONE',  ( 1.511842404626676961, 9.183516746439465805, 1.999999999999998224 ) ) ;
#3052=CARTESIAN_POINT ( 'NONE',  ( 2.406079317367887160, 6.392288322179701332, 1.999999999999998224 ) ) ;
#3053=CARTESIAN_POINT ( 'NONE',  ( 4.683456943470878819, 7.530568860026274791, 13.99999999999999645 ) ) ;
#3062=CARTESIAN_POINT ( 'NONE',  ( -2.440069559021786905, 10.46881825416662259, 13.99999999999999645 ) ) ;
#3067=CARTESIAN_POINT ( 'NONE',  ( -8.013356705133178437, 0.6503825268544297655, 14.00000000000000000 ) ) ;
#3068=CARTESIAN_POINT ( 'NONE',  ( 2.597146444261841491, -5.700021143261159828, 1.999999999999998224 ) ) ;
#3072=CARTESIAN_POINT ( 'NONE',  ( -2.138212235155100061, 7.953261502403491612, 14.00000000000000000 ) ) ;
#3073=EDGE_CURVE ( 'NONE', #2869, #3473, #4302, .T. ) ;
#3077=CARTESIAN_POINT ( 'NONE',  ( -2.965071238690786259, 6.007415411094351398, 13.99999999999999645 ) ) ;
#3080=CARTESIAN_POINT ( 'NONE',  ( 5.612687125617794592, -6.603876269260512188, 1.999999999999998224 ) ) ;
#3081=CARTESIAN_POINT ( 'NONE',  ( 6.824478893064961582, -1.828844244265459329, 1.999999999999998224 ) ) ;
#3084=CARTESIAN_POINT ( 'NONE',  ( 7.108868828250527905, 7.597268273414325535, 1.999999999999998224 ) ) ;
#3086=CARTESIAN_POINT ( 'NONE',  ( 2.389076732465379216, -5.237771676861643577, 1.999999999999998224 ) ) ;
#3092=CARTESIAN_POINT ( 'NONE',  ( 5.279590631142085044, 9.498297537455629325, 13.99999999999999645 ) ) ;
#3097=CARTESIAN_POINT ( 'NONE',  ( -7.945923533235638381, 1.308497053349305883, 14.00000000000000000 ) ) ;
#3098=CARTESIAN_POINT ( 'NONE',  ( -7.375360291558941128, -1.341686286798741135, 1.999999999999998224 ) ) ;
#3101=CARTESIAN_POINT ( 'NONE',  ( 5.059064342543619475, -7.053288479152013402, 14.00000000000000000 ) ) ;
#3104=CARTESIAN_POINT ( 'NONE',  ( 0.7976699882155456889, 9.763020831628287155, 1.999999999999998224 ) ) ;
#3106=CARTESIAN_POINT ( 'NONE',  ( -6.792624376349764681, -3.077375260545992752, 13.99999999999999645 ) ) ;
#3109=CARTESIAN_POINT ( 'NONE',  ( 7.258279873955303607, -6.354128476750924293, 1.999999999999998224 ) ) ;
#3110=CARTESIAN_POINT ( 'NONE',  ( -2.919577271296705412, -6.733962781534540198, 1.999999999999998224 ) ) ;
#3112=UNCERTAINTY_MEASURE_WITH_UNIT (LENGTH_MEASURE( 1.000000000000000082E-05 ), #3372, 'distance_accuracy_value', 'NONE');
#3114=SHAPE_REPRESENTATION_RELATIONSHIP ( 'NONE' , 'NONE' ,  #4116, #1852 ) ;
#3115=FACE_OUTER_BOUND ( 'NONE', #4066, .T. ) ;
#3116=CARTESIAN_POINT ( 'NONE',  ( -3.110890340275366039, -5.031137978950550149, 1.999999999999998224 ) ) ;
#3120=CARTESIAN_POINT ( 'NONE',  ( -10.42442484909544653, -1.371544430045602558, 13.99999999999999645 ) ) ;
#3125=CARTESIAN_POINT ( 'NONE',  ( -8.999716648909560135, -0.5976852874978595409, 14.00000000000000000 ) ) ;
#3126=CARTESIAN_POINT ( 'NONE',  ( 7.937472058416057408, 1.044590838406009414, 1.999999999999998224 ) ) ;
#3127=CARTESIAN_POINT ( 'NONE',  ( -7.301858691287086423, -3.172613069824385068, 1.999999999999998224 ) ) ;
#3128=CARTESIAN_POINT ( 'NONE',  ( -3.231338468933152797, -7.147216519672495494, 14.00000000000000000 ) ) ;
#3130=CARTESIAN_POINT ( 'NONE',  ( 8.697835924490032511, 4.836984431370230375, 1.999999999999998224 ) ) ;
#3133=CARTESIAN_POINT ( 'NONE',  ( 5.806279480218260680, -1.975834710110475401, 13.99999999999999645 ) ) ;
#3135=CARTESIAN_POINT ( 'NONE',  ( -1.271096247112533995, -9.720655361064800104, 1.999999999999998224 ) ) ;
#3136=CARTESIAN_POINT ( 'NONE',  ( -7.375360291558941128, -1.341686286798741135, 1.999999999999998224 ) ) ;
#3140=( NAMED_UNIT ( * ) SI_UNIT ( $, .STERADIAN. ) SOLID_ANGLE_UNIT ( ) );
#3141=CARTESIAN_POINT ( 'NONE',  ( -3.110890340275366039, -5.031137978950550149, 1.999999999999998224 ) ) ;
#3142=CARTESIAN_POINT ( 'NONE',  ( 5.526041665711819206, -0.8982374663919266977, 1.999999999999998224 ) ) ;
#3145=LINE ( 'NONE', #4405, #3191 ) ;
#3146=CARTESIAN_POINT ( 'NONE',  ( -7.660583958272733973, 7.409732212661285011, 13.99999999999999645 ) ) ;
#3152=CARTESIAN_POINT ( 'NONE',  ( 7.258279873954945671, -6.354128476750924293, 14.00000000000000000 ) ) ;
#3153=CARTESIAN_POINT ( 'NONE',  ( 1.183015137239217474, -7.150809911821259135, 1.999999999999998224 ) ) ;
#3155=CARTESIAN_POINT ( 'NONE',  ( 7.716263785693136867, -3.801003699432787375, 1.999999999999998224 ) ) ;
#3156=MECHANICAL_DESIGN_GEOMETRIC_PRESENTATION_REPRESENTATION('',(#1583),#3882);
#3157=CARTESIAN_POINT ( 'NONE',  ( 6.863489721961782308, 6.439594285166703180, 14.00000000000000000 ) ) ;
#3159=CARTESIAN_POINT ( 'NONE',  ( -9.913420430684192652, 3.732070475089103834, 1.999999999999998224 ) ) ;
#3160=CARTESIAN_POINT ( 'NONE',  ( -0.8169484412210609170, 6.196426872864405411, 14.00000000000000000 ) ) ;
#3161=CARTESIAN_POINT ( 'NONE',  ( 5.381714297850043849, -6.137309488907495947, 13.99999999999999645 ) ) ;
#3163=CARTESIAN_POINT ( 'NONE',  ( 7.565999024956893138, -2.848076369834590338, 13.99999999999999645 ) ) ;
#3164=CARTESIAN_POINT ( 'NONE',  ( 5.326024957120313985, -1.813589758486611858, 14.00000000000000000 ) ) ;
#3165=CARTESIAN_POINT ( 'NONE',  ( 8.454926800554316557, -3.338224220245900042, 1.999999999999998224 ) ) ;
#3175=CARTESIAN_POINT ( 'NONE',  ( 1.933011552319069404, 10.64041406927699640, 13.99999999999999645 ) ) ;
#3179=CARTESIAN_POINT ( 'NONE',  ( -7.304208470128496167, 7.056621303512280896, 14.00000000000000000 ) ) ;
#3180=CARTESIAN_POINT ( 'NONE',  ( 6.180183843827202317, 3.174252413088801461, 1.999999999999998224 ) ) ;
#3182=CARTESIAN_POINT ( 'NONE',  ( -7.425829140954076202, 3.215541426300492223, 1.999999999999998224 ) ) ;
#3183=CARTESIAN_POINT ( 'NONE',  ( -6.681386044268952773, 6.252046474378028407, 14.00000000000000000 ) ) ;
#3185=CARTESIAN_POINT ( 'NONE',  ( -4.581738566658409617, -9.288989786611782762, 1.999999999999998224 ) ) ;
#3187=CARTESIAN_POINT ( 'NONE',  ( 8.973806924230895987, -1.178693538871703250, 13.99999999999999645 ) ) ;
#3189=CARTESIAN_POINT ( 'NONE',  ( 2.519353604429575011, -7.832629354751150963, 13.99999999999999645 ) ) ;
#3190=CARTESIAN_POINT ( 'NONE',  ( -2.283612537812034216, 5.775797914528924437, 14.00000000000000000 ) ) ;
#3191=VECTOR ( 'NONE', #1816, 1000.000000000000000 ) ;
#3193=CARTESIAN_POINT ( 'NONE',  ( -5.921118896519414143, 6.318058289644735481, 1.999999999999998224 ) ) ;
#3199=CARTESIAN_POINT ( 'NONE',  ( -5.021280548121167975, 3.603657539922314967, 2.000000000001176392 ) ) ;
#3202=CARTESIAN_POINT ( 'NONE',  ( -3.715337444063474770, -5.771435016728991840, 1.999999999999998224 ) ) ;
#3209=CARTESIAN_POINT ( 'NONE',  ( 9.320190601378300244, -2.164585516638619200, 14.00000000000000000 ) ) ;
#3210=CARTESIAN_POINT ( 'NONE',  ( -5.402835942920797940, -5.063607225391133504, 1.999999999999998224 ) ) ;
#3211=CARTESIAN_POINT ( 'NONE',  ( -6.667513054348624735, -4.302816426345351886, 1.999999999999998224 ) ) ;
#3212=CARTESIAN_POINT ( 'NONE',  ( -9.772156678340820690, -2.119544458102511353, 14.00000000000000000 ) ) ;
#3214=CARTESIAN_POINT ( 'NONE',  ( 5.800093669797941054, -8.375184749302256648, 1.999999999999998224 ) ) ;
#3216=CARTESIAN_POINT ( 'NONE',  ( -8.388197440585694054, -1.387539741535495974, 13.99999999999999645 ) ) ;
#3218=CARTESIAN_POINT ( 'NONE',  ( -0.8169484412210609170, 6.196426872864405411, 14.00000000000000000 ) ) ;
#3220=CARTESIAN_POINT ( 'NONE',  ( -7.884571930971327802, 3.418633173532902969, 1.999999999999998224 ) ) ;
#3223=CARTESIAN_POINT ( 'NONE',  ( -6.876639332705558161, 1.598006320995754237, 1.999999999999998224 ) ) ;
#3225=CARTESIAN_POINT ( 'NONE',  ( 7.439669587982602472, 0.9822684312230360870, 1.999999999999998224 ) ) ;
#3232=CARTESIAN_POINT ( 'NONE',  ( 1.124407659250215685, -9.699258357303232714, 14.00000000000000000 ) ) ;
#3233=CARTESIAN_POINT ( 'NONE',  ( 5.857810772706377733, -5.665644577056675679, 1.999999999999998224 ) ) ;
#3234=CARTESIAN_POINT ( 'NONE',  ( -7.588772809867561087, -4.728083520432016407, 1.999999999999998224 ) ) ;
#3235=CARTESIAN_POINT ( 'NONE',  ( -9.986481889892992569, 1.144076113142371787, 14.00000000000000000 ) ) ;
#3237=ORIENTED_EDGE ( 'NONE', *, *, #5526, .F. ) ;
#3240=CARTESIAN_POINT ( 'NONE',  ( 1.598519525623709692, 9.677660462521252782, 13.99999999999999645 ) ) ;
#3243=CARTESIAN_POINT ( 'NONE',  ( 4.513069810084764377, -3.445129632735343339, 14.00000000000000000 ) ) ;
#3245=CARTESIAN_POINT ( 'NONE',  ( 1.208067634251008604, -9.180948453718620783, 1.999999999999998224 ) ) ;
#3248=CARTESIAN_POINT ( 'NONE',  ( -6.334648143026943679, -2.872559841353752308, 1.999999999999998224 ) ) ;
#3251=CARTESIAN_POINT ( 'NONE',  ( 7.097632634466812362, -2.668286824979932970, 1.999999999999998224 ) ) ;
#3261=CARTESIAN_POINT ( 'NONE',  ( 5.030817567586885808, 9.062633982223131213, 14.00000000000000000 ) ) ;
#3262=CARTESIAN_POINT ( 'NONE',  ( 8.952336951391263398, 1.032601321559316832, 1.999999999999998224 ) ) ;
#3264=CARTESIAN_POINT ( 'NONE',  ( -2.970508497641843881, 8.737606122598624125, 1.999999999999998224 ) ) ;
#3265=CARTESIAN_POINT ( 'NONE',  ( 5.710084532570044225, 7.448680193042861220, 14.00000000000000000 ) ) ;
#3271=CARTESIAN_POINT ( 'NONE',  ( 8.697835924490034287, 4.836984431370582982, 13.99999999999999645 ) ) ;
#3272=VECTOR ( 'NONE', #1678, 1000.000000000000000 ) ;
#3273=CARTESIAN_POINT ( 'NONE',  ( -3.987231204388229422, 4.693390172674912542, 13.99999999999953104 ) ) ;
#3275=CARTESIAN_POINT ( 'NONE',  ( -5.390757458300977412, 6.793134358447004750, 1.999999999999998224 ) ) ;
#3279=CARTESIAN_POINT ( 'NONE',  ( 4.815977876496239318, 4.225366587634176163, 1.999999999999998224 ) ) ;
#3281=CARTESIAN_POINT ( 'NONE',  ( -4.089163901200156381, 5.898691170885093982, 1.999999999999998224 ) ) ;
#3292=CARTESIAN_POINT ( 'NONE',  ( 6.401046915551857452, 6.194151307162986342, 1.999999999999998224 ) ) ;
#3294=CARTESIAN_POINT ( 'NONE',  ( 6.444084565535373343, 4.617298776321548281, 13.99999999999999645 ) ) ;
#3295=CARTESIAN_POINT ( 'NONE',  ( 9.164356920907600568, 2.464151434936005192, 1.999999999999998224 ) ) ;
#3296=CARTESIAN_POINT ( 'NONE',  ( -9.445900372710701376, 3.550092993115766760, 14.00000000000000000 ) ) ;
#3301=CARTESIAN_POINT ( 'NONE',  ( -4.184906021401652687, -5.457255036755483069, 14.00000000000000000 ) ) ;
#3302=CARTESIAN_POINT ( 'NONE',  ( 5.347643153870340171, -7.463670412150953837, 13.99999999999999645 ) ) ;
#3303=CARTESIAN_POINT ( 'NONE',  ( 2.161943361801395014, -6.363123982928430067, 14.00000000000000000 ) ) ;
#3305=CARTESIAN_POINT ( 'NONE',  ( -9.742306995815773973, -3.848972158781406083, 1.999999999999998224 ) ) ;
#3308=CARTESIAN_POINT ( 'NONE',  ( -2.189112655477410740, -6.464091385745793339, 1.999999999999998224 ) ) ;
#3310=CARTESIAN_POINT ( 'NONE',  ( 5.772253124442284111, -3.205917188174072230, 1.999999999999998224 ) ) ;
#3320=CARTESIAN_POINT ( 'NONE',  ( -0.3010823416051299772, -9.281161307073867661, 1.999999999999998224 ) ) ;
#3322=CARTESIAN_POINT ( 'NONE',  ( -3.594774944545354955, 7.935102286574237773, 13.99999999999999645 ) ) ;
#3323=CARTESIAN_POINT ( 'NONE',  ( 10.50003631213658117, 0.006025845833179007717, 14.00000000000000000 ) ) ;
#3324=VERTEX_POINT ( 'NONE', #2657 ) ;
#3327=CARTESIAN_POINT ( 'NONE',  ( 10.40193138080405255, 3.529992181067783452, 1.999999999999998224 ) ) ;
#3328=CARTESIAN_POINT ( 'NONE',  ( 7.280083392764700179, -2.072676875633882254, 14.00000000000000000 ) ) ;
#3329=CARTESIAN_POINT ( 'NONE',  ( -8.402144917908875854, 4.670158400850172420, 13.99999999999999645 ) ) ;
#3331=CARTESIAN_POINT ( 'NONE',  ( -1.987635485262058577, 6.951293809708866789, 14.00000000000000000 ) ) ;
#3333=CARTESIAN_POINT ( 'NONE',  ( -7.945634105012028492, -6.745245841440164369, 1.999999999999998224 ) ) ;
#3337=CARTESIAN_POINT ( 'NONE',  ( -5.395431796987671724, -5.765308706272893602, 1.999999999999998224 ) ) ;
#3339=CARTESIAN_POINT ( 'NONE',  ( -2.020383375745208987, -7.552201994671270846, 1.999999999999998224 ) ) ;
#3340=CARTESIAN_POINT ( 'NONE',  ( -0.4015567206217142693, -6.330257989742454683, 1.999999999999998224 ) ) ;
#3341=CARTESIAN_POINT ( 'NONE',  ( 3.426039378954557346, 5.938690629332270987, 13.99999999999999645 ) ) ;
#3348=CARTESIAN_POINT ( 'NONE',  ( -1.484422800923325125, -8.172499773499277254, 1.999999999999998224 ) ) ;
#3350=CARTESIAN_POINT ( 'NONE',  ( 7.132151089625189400, 3.519983721611798622, 13.99999999999999645 ) ) ;
#3357=CARTESIAN_POINT ( 'NONE',  ( 7.097632634466814139, -2.668286824980076855, 14.00000000000000000 ) ) ;
#3358=CARTESIAN_POINT ( 'NONE',  ( -5.250997584835957355, 8.145342823909338392, 13.99999999999999645 ) ) ;
#3361=CARTESIAN_POINT ( 'NONE',  ( 4.815977876496241095, 4.225366587634054483, 14.00000000000000000 ) ) ;
#3363=CARTESIAN_POINT ( 'NONE',  ( 6.019515613300546519, 7.843576796802394391, 1.999999999999998224 ) ) ;
#3367=CARTESIAN_POINT ( 'NONE',  ( -6.453089103408601090, 4.947336467533990145, 1.999999999999998224 ) ) ;
#3369=CARTESIAN_POINT ( 'NONE',  ( 6.026041665150464688, -0.9817477132364114123, 1.999999999999998224 ) ) ;
#3370=CARTESIAN_POINT ( 'NONE',  ( -0.8811140424828162176, 6.693995663234412419, 13.99999999999999645 ) ) ;
#3372=( LENGTH_UNIT ( ) NAMED_UNIT ( * ) SI_UNIT ( .MILLI., .METRE. ) );
#3379=CARTESIAN_POINT ( 'NONE',  ( -9.406456921418630657, 1.708717176649225511, 1.999999999999998224 ) ) ;
#3381=CARTESIAN_POINT ( 'NONE',  ( 9.077580196901687160, 4.112174628513754371, 13.99999999999999645 ) ) ;
#3383=ORIENTED_EDGE ( 'NONE', *, *, #4034, .T. ) ;
#3388=CARTESIAN_POINT ( 'NONE',  ( 6.523553822664519330, -0.1051741892335816969, 14.00000000000000000 ) ) ;
#3389=CARTESIAN_POINT ( 'NONE',  ( -4.310533329768688304, 5.077046166951620698, 1.999999999999412914 ) ) ;
#3390=CARTESIAN_POINT ( 'NONE',  ( -5.034899347480884302, -4.722558430572732391, 14.00000000000000000 ) ) ;
#3393=CARTESIAN_POINT ( 'NONE',  ( 8.595497693523489247, -5.345940745659027549, 1.999999999999998224 ) ) ;
#3396=CARTESIAN_POINT ( 'NONE',  ( 6.592258996018686368, -3.799026305082465971, 1.999999999999998224 ) ) ;
#3398=CARTESIAN_POINT ( 'NONE',  ( -2.721086536275892254, 7.222755814214462333, 13.99999999999999645 ) ) ;
#3399=B_SPLINE_SURFACE_WITH_KNOTS ( 'NONE', 1, 3, ( 
 ( #1752, #5296, #1356, #919, #4427, #482, #2241, #1811, #3570, #3141, #4888, #2270, #3654, #1865, #5462, #1519, #3199, #2848, #1087, #4117, #3622, #170, #4969, #2785, #5381, #1116, #226, #5408, #2873, #4570, #3279, #1466, #4946, #631, #2295, #4055, #5031, #2819, #1004, #1439, #5493, #2763, #2382, #1488, #4141, #4626, #566, #4600, #1555, #108, #600, #3308, #4515, #2322, #1980, #4171, #4084, #3677, #3248, #195, #5058, #137, #1896, #3223, #1027, #2409, #4541, #2350, #1922, #3735, #659, #5433, #4997, #1057, #1948, #3702, #4202, #2066, #3853, #2440, #5579, #1640, #3766, #253, #5520, #2556, #1207, #1180, #2931, #5171, #366, #3396, #3878, #3793, #4229, #688, #1578, #2495, #3445, #5633, #1690, #4656, #4317, #5149, #5204, #2124, #3337, #1145, #2471, #4683, #2095, #1263, #3823, #3025, #2012, #280, #2959, #4708, #3367, #5088, #4254, #771, #2903, #1232, #722, #2037, #5550, #1607, #5122, #743, #2521, #4285, #339, #305, #5605, #1664, #3420, #2991, #4737, #803, #2645, #3531, #49, #2264, #3591, #3080, #4023, #3906, #3476, #2694, #939, #5663, #453, #22, #913, #79, #2153, #2582, #425, #4341, #4883, #2183, #5263, #392, #508, #1804, #4450, #1834, #885, #5344, #1724, #5238, #2212, #2234, #830, #3963, #1775, #1294, #3051, #4795, #1402, #5292, #1318, #4824, #3563, #4769, #1349, #856, #3938, #2612, #4371, #2415, #4398, #1748, #3503, #3109, #4857, #2671, #4423, #476, #3990, #5320, #1379, #3135, #3646, #4562, #218, #592, #1975, #1081, #2757, #4535, #5429, #131, #3728, #4965, #2344, #4912, #3697, #2843, #1861, #970, #4510, #4595, #654, #4110, #1918, #164, #2404, #3673, #626, #2317, #4941, #5487, #1461, #1023, #1484, #2376, #4136, #4050, #5455, #1944 ),
 ( #4165, #562, #3164, #3243, #191, #4077, #104, #4990, #2728, #4481, #1511, #1050, #3617, #539, #2290, #5375, #2811, #3273, #5024, #1431, #3190, #999, #3218, #2781, #1890, #5403, #765, #2434, #2090, #332, #3361, #1111, #5115, #4223, #2033, #4621, #361, #5166, #2897, #2117, #3818, #2515, #716, #4196, #5572, #1549, #3303, #4280, #2057, #245, #2868, #4731, #2007, #1632, #738, #3390, #3873, #5515, #3848, #796, #5053, #5543, #2549, #680, #3759, #1227, #3414, #1574, #2925, #2492, #5142, #4310, #3331, #5082, #4649, #1137, #1659, #2466, #3788, #275, #2983, #5600, #1600, #1171, #4677, #4248, #299, #1201, #2951, #4703, #1684, #4816, #879, #3018, #3440, #4763, #1798, #448, #419, #2177, #4416, #5313, #2638, #3128, #3044, #3471, #5625, #824, #1743, #2687, #4877, #933, #3900, #3553, #4392, #4443, #1373, #2577, #386, #1718, #3933, #1341, #498, #3072, #2257, #5198, #5232, #1313, #2205, #2605, #1257, #3498, #3957, #4335, #470, #2146, #5657, #1289, #4789, #849, #4363, #16, #1767, #3523, #5685, #5285, #3101, #5257, #4849, #906, #2665, #2229, #3982, #42, #4014, #2836, #4933, #98, #2283, #3691, #2337, #4043, #584, #1854, #992, #5448, #2370, #4103, #3611, #1424, #3183, #4588, #157, #4130, #1478, #5422, #1882, #71, #1456, #1396, #4960, #1502, #3265, #3157, #963, #1913, #1827, #2720, #5016, #1074, #3585, #646, #1042, #616, #3668, #184, #4903, #5338, #1017, #4503, #5366, #2751, #1937, #2803, #556, #4472, #2311, #4071, #532, #123, #3640, #4555, #5396, #3212, #2775, #4530, #3235, #4983, #3296, #2973, #2484, #2507, #5563, #3780, #4240, #2049, #3807, #5159, #3407, #1129, #1591, #2860, #266, #1219, #5592, #4186, #321, #1652, #291, #1193, #1624, #3323 ) ),
 .UNSPECIFIED., .F., .F., .F.,
 ( 2, 2 ),
 ( 4, 2, 2, 2, 2, 2, 2, 2, 2, 2, 2, 2, 2, 2, 2, 2, 2, 2, 2, 2, 2, 2, 2, 2, 2, 2, 2, 2, 2, 2, 2, 2, 2, 2, 2, 2, 2, 2, 2, 2, 2, 2, 2, 2, 2, 2, 2, 2, 2, 2, 2, 2, 2, 2, 2, 2, 2, 2, 2, 2, 2, 2, 2, 2, 2, 2, 2, 2, 2, 2, 2, 2, 2, 2, 2, 2, 2, 2, 2, 2, 2, 2, 2, 2, 2, 2, 2, 2, 2, 2, 2, 2, 2, 2, 2, 2, 2, 2, 2, 2, 2, 2, 2, 2, 2, 2, 2, 2, 2, 2, 2, 2, 2, 2, 2, 2, 2, 2, 2, 2, 4 ),
 ( 0.5000000000000000000, 0.9800000000000000933 ),
 ( 0.000000000000000000, 0.01562500000000000000, 0.03125000000000000000, 0.04687500000000000000, 0.06250000000000000000, 0.07812500000000000000, 0.09375000000000000000, 0.1093750000000000000, 0.1250000000000000000, 0.1328125000000000000, 0.1406250000000000000, 0.1484375000000000000, 0.1562500000000000000, 0.1640625000000000000, 0.1718750000000000000, 0.1796875000000000000, 0.1875000000000000000, 0.1953125000000000000, 0.2031250000000000000, 0.2109375000000000000, 0.2187500000000000000, 0.2265625000000000000, 0.2343750000000000000, 0.2421875000000000000, 0.2500000000000000000, 0.2578125000000000000, 0.2656250000000000000, 0.2734375000000000000, 0.2812500000000000000, 0.2890625000000000000, 0.2968750000000000000, 0.3046875000000000000, 0.3125000000000000000, 0.3203125000000000000, 0.3281250000000000000, 0.3359375000000000000, 0.3437500000000000000, 0.3515625000000000000, 0.3593750000000000000, 0.3671875000000000000, 0.3750000000000000000, 0.3828125000000000000, 0.3906250000000000000, 0.3984375000000000000, 0.4062500000000000000, 0.4140625000000000000, 0.4218750000000000000, 0.4296875000000000000, 0.4375000000000000000, 0.4453125000000000000, 0.4531250000000000000, 0.4609375000000000000, 0.4687500000000000000, 0.4765625000000000000, 0.4843750000000000000, 0.4921875000000000000, 0.5000000000000000000, 0.5078125000000000000, 0.5156250000000000000, 0.5234375000000000000, 0.5312500000000000000, 0.5390625000000000000, 0.5468750000000000000, 0.5546875000000000000, 0.5625000000000000000, 0.5703125000000000000, 0.5781250000000000000, 0.5859375000000000000, 0.5937500000000000000, 0.6015625000000000000, 0.6093750000000000000, 0.6171875000000000000, 0.6250000000000000000, 0.6328125000000000000, 0.6406250000000000000, 0.6484375000000000000, 0.6562500000000000000, 0.6640625000000000000, 0.6718750000000000000, 0.6796875000000000000, 0.6875000000000000000, 0.6953125000000000000, 0.7031250000000000000, 0.7109375000000000000, 0.7187500000000000000, 0.7265625000000000000, 0.7343750000000000000, 0.7421875000000000000, 0.7500000000000000000, 0.7578125000000000000, 0.7656250000000000000, 0.7734375000000000000, 0.7812500000000000000, 0.7890625000000000000, 0.7968750000000000000, 0.8046875000000000000, 0.8125000000000000000, 0.8203125000000000000, 0.8281250000000000000, 0.8359375000000000000, 0.8437500000000000000, 0.8515625000000000000, 0.8593750000000000000, 0.8671875000000000000, 0.8750000000000000000, 0.8828125000000000000, 0.8906250000000000000, 0.8984375000000000000, 0.9062500000000000000, 0.9140625000000000000, 0.9218750000000000000, 0.9296875000000000000, 0.9375000000000000000, 0.9453125000000000000, 0.9531250000000000000, 0.9609375000000000000, 0.9687500000000000000, 0.9765625000000000000, 0.9843750000000000000, 0.9921875000000000000, 1.000000000000000000 ),
 .UNSPECIFIED. ) ;
#3400=CARTESIAN_POINT ( 'NONE',  ( 7.379526280503348801, 5.862399640741291051, 1.999999999999998224 ) ) ;
#3406=CARTESIAN_POINT ( 'NONE',  ( -0.1462562576243747192, 8.775315755192165668, 13.99999999999999645 ) ) ;
#3407=CARTESIAN_POINT ( 'NONE',  ( 0.1634456542307747284, 10.28566380800474889, 14.00000000000000000 ) ) ;
#3412=CARTESIAN_POINT ( 'NONE',  ( -5.416162817796315920, -4.301262981183149314, 14.00000000000000000 ) ) ;
#3413=CARTESIAN_POINT ( 'NONE',  ( -4.892757975385814362, 9.527326283048992650, 13.99999999999999645 ) ) ;
#3414=CARTESIAN_POINT ( 'NONE',  ( -6.041022033915573353, 3.753782041847178341, 14.00000000000000000 ) ) ;
#3415=ORIENTED_EDGE ( 'NONE', *, *, #3073, .T. ) ;
#3417=CARTESIAN_POINT ( 'NONE',  ( -7.551678268146208239, 5.989845445213456188, 1.999999999999998224 ) ) ;
#3420=CARTESIAN_POINT ( 'NONE',  ( 8.156937663705429387, 2.333191796391003603, 1.999999999999998224 ) ) ;
#3421=CARTESIAN_POINT ( 'NONE',  ( -6.576488680450179203, -0.2289623203888876135, 1.999999999999998224 ) ) ;
#3422=CARTESIAN_POINT ( 'NONE',  ( 6.638644669766899931, 2.135480210976827831, 13.99999999999999645 ) ) ;
#3424=CARTESIAN_POINT ( 'NONE',  ( -2.331745755519268215, 9.978964459600444314, 1.999999999999998224 ) ) ;
#3430=CARTESIAN_POINT ( 'NONE',  ( 1.208067634251009270, -9.180948453718622559, 13.99999999999999645 ) ) ;
#3436=CARTESIAN_POINT ( 'NONE',  ( -5.395431796987672612, -5.765308706272596950, 14.00000000000000000 ) ) ;
#3437=CARTESIAN_POINT ( 'NONE',  ( -10.17357856257779680, 2.902115915870757679, 13.99999999999999645 ) ) ;
#3440=CARTESIAN_POINT ( 'NONE',  ( 5.053476174606819527, -5.757900651972699180, 14.00000000000000000 ) ) ;
#3442=VERTEX_POINT ( 'NONE', #550 ) ;
#3443=CARTESIAN_POINT ( 'NONE',  ( -9.913420430684192652, 3.732070475089103834, 1.999999999999998224 ) ) ;
#3444=CARTESIAN_POINT ( 'NONE',  ( 6.460119401626726265, -2.924461030940389783, 13.99999999999999645 ) ) ;
#3445=CARTESIAN_POINT ( 'NONE',  ( 1.760389272475360256, -7.536528230137968798, 1.999999999999998224 ) ) ;
#3447=CARTESIAN_POINT ( 'NONE',  ( -5.322107489685387272, 5.499660323246577498, 13.99999999999999645 ) ) ;
#3451=CARTESIAN_POINT ( 'NONE',  ( 0.3244988297792679166, -9.772062696132405080, 1.999999999999998224 ) ) ;
#3458=CARTESIAN_POINT ( 'NONE',  ( 5.348203032363755050, 8.300083771889282147, 13.99999999999999645 ) ) ;
#3461=CARTESIAN_POINT ( 'NONE',  ( 6.000000000000000000, 0.000000000000000000, 1.999999999999998224 ) ) ;
#3467=CARTESIAN_POINT ( 'NONE',  ( 3.857245400775171529, -7.804869966781184054, 14.00000000000000000 ) ) ;
#3468=CARTESIAN_POINT ( 'NONE',  ( 4.243312049792013596, -4.537448458213932945, 1.999999999999998224 ) ) ;
#3471=CARTESIAN_POINT ( 'NONE',  ( -4.895455514773497718, -6.178604150901620073, 14.00000000000000000 ) ) ;
#3473=VERTEX_POINT ( 'NONE', #3772 ) ;
#3475=CARTESIAN_POINT ( 'NONE',  ( 2.406079317367887604, 6.392288322179703108, 13.99999999999999645 ) ) ;
#3476=CARTESIAN_POINT ( 'NONE',  ( 3.208073253695059801, -8.107602109809695534, 1.999999999999998224 ) ) ;
#3477=CARTESIAN_POINT ( 'NONE',  ( 7.992346231215205599, -0.9198489573344823533, 1.999999999999998224 ) ) ;
#3478=CARTESIAN_POINT ( 'NONE',  ( -4.227552200850896114, 7.601683304540504338, 13.99999999999999645 ) ) ;
#3486=CARTESIAN_POINT ( 'NONE',  ( -3.290073422422831406, -8.739709727799914063, 13.99999999999999645 ) ) ;
#3494=CARTESIAN_POINT ( 'NONE',  ( 8.518575158374426692, 0.2826087140540691767, 14.00000000000000000 ) ) ;
#3496=CARTESIAN_POINT ( 'NONE',  ( 1.933011552319069404, 10.64041406927699640, 13.99999999999999645 ) ) ;
#3498=CARTESIAN_POINT ( 'NONE',  ( 5.528193227149303723, 6.314447692498919018, 14.00000000000000000 ) ) ;
#3501=CARTESIAN_POINT ( 'NONE',  ( -4.256527737016168267, -4.845957569453232416, 13.99999999999999645 ) ) ;
#3503=CARTESIAN_POINT ( 'NONE',  ( 8.172274133037948474, -5.076547540501181288, 1.999999999999998224 ) ) ;
#3505=CARTESIAN_POINT ( 'NONE',  ( -5.745624475482103755, 5.035517847229626476, 1.999999999999998224 ) ) ;
#3513=CARTESIAN_POINT ( 'NONE',  ( 11.00000000000000355, -2.488243985854232676E-14, 13.99999999999999645 ) ) ;
#3517=CARTESIAN_POINT ( 'NONE',  ( 2.597146444261842824, -5.700021143261160717, 13.99999999999999645 ) ) ;
#3520=CARTESIAN_POINT ( 'NONE',  ( -3.231338468933152797, -7.147216519672495494, 14.00000000000000000 ) ) ;
#3521=CARTESIAN_POINT ( 'NONE',  ( 6.460119401626724489, -2.924461030940388895, 1.999999999999998224 ) ) ;
#3523=CARTESIAN_POINT ( 'NONE',  ( 7.017208779832877497, -5.019401656905778886, 14.00000000000000000 ) ) ;
#3525=CARTESIAN_POINT ( 'NONE',  ( -5.250997584835956467, 8.145342823910020513, 1.999999999999998224 ) ) ;
#3528=CARTESIAN_POINT ( 'NONE',  ( 2.321214644803172522, -6.838859567843808662, 13.99999999999999645 ) ) ;
#3531=CARTESIAN_POINT ( 'NONE',  ( 7.990059919442647818, -3.149571442993177595, 1.999999999999998224 ) ) ;
#3532=CARTESIAN_POINT ( 'NONE',  ( 6.804422688527091978, 1.586354726853912434, 1.999999999999998224 ) ) ;
#3538=CARTESIAN_POINT ( 'NONE',  ( 3.173694703385744997, 5.505084763670540227, 1.999999999999998224 ) ) ;
#3543=CARTESIAN_POINT ( 'NONE',  ( 10.40193138080327628, 3.529992181067589829, 13.99999999999999645 ) ) ;
#3549=CARTESIAN_POINT ( 'NONE',  ( -7.986673696634112751, -0.6581801297105769333, 14.00000000000000000 ) ) ;
#3550=CARTESIAN_POINT ( 'NONE',  ( 3.471913601335177013, 7.039518430846525732, 1.999999999999998224 ) ) ;
#3553=CARTESIAN_POINT ( 'NONE',  ( -8.013356705133178437, 0.6503825268544297655, 14.00000000000000000 ) ) ;
#3557=CARTESIAN_POINT ( 'NONE',  ( -7.945634105012028492, -6.745245841440164369, 1.999999999999998224 ) ) ;
#3558=CARTESIAN_POINT ( 'NONE',  ( 5.500000000000001776, 0.000000000000000000, 14.00000000000000000 ) ) ;
#3559=CARTESIAN_POINT ( 'NONE',  ( 6.824478893064963358, -1.828844244265460217, 13.99999999999999645 ) ) ;
#3563=CARTESIAN_POINT ( 'NONE',  ( 7.379526280503348801, 5.862399640741291051, 1.999999999999998224 ) ) ;
#3564=CARTESIAN_POINT ( 'NONE',  ( -6.465640026559585252, 4.020973141381892546, 1.999999999999998224 ) ) ;
#3567=EDGE_CURVE ( 'NONE', #3442, #3843, #1153, .T. ) ;
#3570=CARTESIAN_POINT ( 'NONE',  ( -1.336592501075286599, -5.709464570123371274, 1.999999999999998224 ) ) ;
#3571=CARTESIAN_POINT ( 'NONE',  ( 5.326024957120312209, -1.813589758486610970, 1.999999999999998224 ) ) ;
#3575=CARTESIAN_POINT ( 'NONE',  ( 0.1774200004017887078, 10.78715707688374614, 13.99999999999999645 ) ) ;
#3580=EDGE_CURVE ( 'NONE', #3473, #261, #178, .T. ) ;
#3582=CARTESIAN_POINT ( 'NONE',  ( 4.853468040355885194, -8.397360160973688537, 14.00000000000000000 ) ) ;
#3583=CARTESIAN_POINT ( 'NONE',  ( -3.989331152809321157, -6.191695749071041810, 1.999999999999998224 ) ) ;
#3584=CARTESIAN_POINT ( 'NONE',  ( 8.453438707198472457, 0.9797652757261496870, 1.999999999999998224 ) ) ;
#3585=CARTESIAN_POINT ( 'NONE',  ( 9.522148329495834673, -0.6196525284526704924, 14.00000000000000000 ) ) ;
#3587=CARTESIAN_POINT ( 'NONE',  ( 6.019515613300546519, 7.843576796802394391, 1.999999999999998224 ) ) ;
#3589=CARTESIAN_POINT ( 'NONE',  ( 7.761517335261691741, -2.213789340049631349, 13.99999999999999645 ) ) ;
#3590=CARTESIAN_POINT ( 'NONE',  ( -2.721086536275892254, 7.222755814214462333, 13.99999999999999645 ) ) ;
#3591=CARTESIAN_POINT ( 'NONE',  ( 6.591354251721933011, -5.587324598951576071, 1.999999999999998224 ) ) ;
#3593=CARTESIAN_POINT ( 'NONE',  ( -5.810612947751084612, -4.611264106266946605, 1.999999999999998224 ) ) ;
#3594=( LENGTH_UNIT ( ) NAMED_UNIT ( * ) SI_UNIT ( .MILLI., .METRE. ) );
#3601=CARTESIAN_POINT ( 'NONE',  ( 2.810994617404221962, -9.846529629020569274, 13.99999999999999645 ) ) ;
#3606=COLOUR_RGB ( '',0.8941176470588234615, 0.8941176470588234615, 0.8941176470588234615 ) ;
#3607=CARTESIAN_POINT ( 'NONE',  ( 5.710084532570044225, 7.448680193042861220, 14.00000000000000000 ) ) ;
#3608=CARTESIAN_POINT ( 'NONE',  ( 6.804422688527091978, 1.586354726853912434, 1.999999999999998224 ) ) ;
#3609=CARTESIAN_POINT ( 'NONE',  ( 6.591354251721933011, -5.587324598951576071, 1.999999999999998224 ) ) ;
#3611=CARTESIAN_POINT ( 'NONE',  ( -7.966005157978615969, 4.422220743486623640, 14.00000000000000000 ) ) ;
#3613=CARTESIAN_POINT ( 'NONE',  ( -0.7976699882155984245, 9.736979168371712845, 1.999999999999998224 ) ) ;
#3615=CARTESIAN_POINT ( 'NONE',  ( 8.396466517618241809, 3.163083589105052607, 13.99999999999999645 ) ) ;
#3616=CARTESIAN_POINT ( 'NONE',  ( -8.513020831365363250, 0.6954046021538080602, 13.99999999999999645 ) ) ;
#3617=CARTESIAN_POINT ( 'NONE',  ( -5.637968025906140213, -2.116521738900702942, 14.00000000000000000 ) ) ;
#3618=CARTESIAN_POINT ( 'NONE',  ( 7.344045208304290639, 5.086154276871864610, 1.999999999999998224 ) ) ;
#3622=CARTESIAN_POINT ( 'NONE',  ( -2.283612537812033771, 5.775797914528922661, 1.999999999999998224 ) ) ;
#3627=CARTESIAN_POINT ( 'NONE',  ( -4.256527737016168267, -4.845957569453232416, 13.99999999999999645 ) ) ;
#3632=ORIENTED_EDGE ( 'NONE', *, *, #2172, .T. ) ;
#3635=CARTESIAN_POINT ( 'NONE',  ( -6.681386044268952773, 6.252046474378028407, 14.00000000000000000 ) ) ;
#3636=CARTESIAN_POINT ( 'NONE',  ( 5.586635445632133212, -4.430858740432559451, 1.999999999999998224 ) ) ;
#3639=CARTESIAN_POINT ( 'NONE',  ( -7.945923533235636604, 1.308497053349305439, 1.999999999999998224 ) ) ;
#3640=CARTESIAN_POINT ( 'NONE',  ( -8.072272399573057200, -5.790267008922743486, 14.00000000000000000 ) ) ;
#3642=CARTESIAN_POINT ( 'NONE',  ( 2.803319092186594030, 10.45862564946446760, 1.999999999999998224 ) ) ;
#3643=CARTESIAN_POINT ( 'NONE',  ( -5.183646570197097958, -3.010418922386785212, 14.00000000000000000 ) ) ;
#3644=CARTESIAN_POINT ( 'NONE',  ( 7.812003909081977504, 1.689803927524662797, 13.99999999999999645 ) ) ;
#3646=CARTESIAN_POINT ( 'NONE',  ( -2.067895747887561697, -9.596367745172036834, 1.999999999999998224 ) ) ;
#3649=CARTESIAN_POINT ( 'NONE',  ( 0.5432484998931219611, -8.249156888542632515, 1.999999999999998224 ) ) ;
#3654=CARTESIAN_POINT ( 'NONE',  ( -5.637968025906138436, -2.116521738900817073, 1.999999999999998224 ) ) ;
#3657=CARTESIAN_POINT ( 'NONE',  ( 6.680730669075649608, 3.301097878975988387, 1.999999999999998224 ) ) ;
#3662=CARTESIAN_POINT ( 'NONE',  ( 10.75001815606828970, 0.003012922916577078902, 14.00000000000000000 ) ) ;
#3665=CARTESIAN_POINT ( 'NONE',  ( 6.721134410589271191, -6.938257756002876420, 14.00000000000000000 ) ) ;
#3666=CARTESIAN_POINT ( 'NONE',  ( -5.210352092881994857, -6.569156856910357334, 1.999999999999998224 ) ) ;
#3667=CARTESIAN_POINT ( 'NONE',  ( -7.652305818843809782, 2.590529227167489790, 1.999999999999998224 ) ) ;
#3668=CARTESIAN_POINT ( 'NONE',  ( 8.172274133038307298, -5.076547540501183065, 14.00000000000000000 ) ) ;
#3671=CARTESIAN_POINT ( 'NONE',  ( 3.173694703385745886, 5.505084763670784476, 14.00000000000000000 ) ) ;
#3672=CARTESIAN_POINT ( 'NONE',  ( 9.020117466465418232, 0.2947087185667972564, 13.99999999999999645 ) ) ;
#3673=CARTESIAN_POINT ( 'NONE',  ( 1.837295235934470305, 10.14794156482770049, 1.999999999999998224 ) ) ;
#3675=CARTESIAN_POINT ( 'NONE',  ( 4.043470907200509501, 7.877814422643418801, 1.999999999999998224 ) ) ;
#3677=CARTESIAN_POINT ( 'NONE',  ( -6.065725208710914806, -3.376743199310592747, 1.999999999999998224 ) ) ;
#3680=CARTESIAN_POINT ( 'NONE',  ( 2.672042568001582019, -6.151894458593051063, 1.999999999999998224 ) ) ;
#3688=CARTESIAN_POINT ( 'NONE',  ( 6.863489721961782308, 6.439594285166703180, 14.00000000000000000 ) ) ;
#3689=CARTESIAN_POINT ( 'NONE',  ( 8.640499015841685448, 2.466831329604985079, 1.999999999999998224 ) ) ;
#3690=CARTESIAN_POINT ( 'NONE',  ( -3.109042548464319378, -8.271822080922653697, 1.999999999999998224 ) ) ;
#3691=CARTESIAN_POINT ( 'NONE',  ( -7.588772809867895930, -4.728083520431684228, 14.00000000000000000 ) ) ;
#3696=CARTESIAN_POINT ( 'NONE',  ( -3.798941939731700579, -9.621416145859109648, 13.99999999999999645 ) ) ;
#3697=CARTESIAN_POINT ( 'NONE',  ( -9.445900372709948201, 3.550092993115765871, 1.999999999999998224 ) ) ;
#3699=CARTESIAN_POINT ( 'NONE',  ( -8.513020831365363250, 0.6954046021538080602, 1.999999999999998224 ) ) ;
#3702=CARTESIAN_POINT ( 'NONE',  ( 0.9466184546083533657, 7.233353930637701268, 1.999999999999998224 ) ) ;
#3704=CARTESIAN_POINT ( 'NONE',  ( 3.621982275015807051, -5.614208739972523787, 1.999999999999998224 ) ) ;
#3714=CARTESIAN_POINT ( 'NONE',  ( 5.347643153870339283, -7.463670412152253242, 1.999999999999998224 ) ) ;
#3716=CARTESIAN_POINT ( 'NONE',  ( 1.649120185255091187, 7.633850905136058351, 13.99999999999999645 ) ) ;
#3718=CARTESIAN_POINT ( 'NONE',  ( -6.708753103182418798, 7.642576097240645794, 1.999999999999998224 ) ) ;
#3725=CARTESIAN_POINT ( 'NONE',  ( -6.041022033915573353, 3.753782041847178341, 14.00000000000000000 ) ) ;
#3726=CARTESIAN_POINT ( 'NONE',  ( -3.867583043141954224, 8.914321633329153727, 13.99999999999999645 ) ) ;
#3728=CARTESIAN_POINT ( 'NONE',  ( -9.926332099420363875, -1.311590842189569894, 1.999999999999998224 ) ) ;
#3731=CARTESIAN_POINT ( 'NONE',  ( -9.533152408061617678, 0.1566715252477025866, 1.999999999999998224 ) ) ;
#3735=CARTESIAN_POINT ( 'NONE',  ( -4.089163901200156381, 5.898691170885093982, 1.999999999999998224 ) ) ;
#3737=CARTESIAN_POINT ( 'NONE',  ( 1.103627080440590102, -6.655442145117440589, 1.999999999999998224 ) ) ;
#3748=CARTESIAN_POINT ( 'NONE',  ( -0.6809175113353355124, 10.25113960786383949, 14.00000000000000000 ) ) ;
#3749=CARTESIAN_POINT ( 'NONE',  ( 1.999247522871089311, 8.586038698136235325, 1.999999999999998224 ) ) ;
#3750=CARTESIAN_POINT ( 'NONE',  ( -7.519441789400338472, 0.4931591957933217363, 13.99999999999999645 ) ) ;
#3757=CARTESIAN_POINT ( 'NONE',  ( 6.034497645749724803, 4.327592090611794617, 14.00000000000000000 ) ) ;
#3758=CARTESIAN_POINT ( 'NONE',  ( 9.650319724629330409, 2.588775111615905011, 13.99999999999999645 ) ) ;
#3759=CARTESIAN_POINT ( 'NONE',  ( -6.734745854536168252, 2.161492950162117399, 14.00000000000000000 ) ) ;
#3762=CARTESIAN_POINT ( 'NONE',  ( -5.893815055328603947, 7.676334994785346311, 1.999999999999998224 ) ) ;
#3766=CARTESIAN_POINT ( 'NONE',  ( 6.034497645749723027, 4.327592090611793729, 1.999999999999998224 ) ) ;
#3768=CARTESIAN_POINT ( 'NONE',  ( 4.776808680784692562, 5.634249062854761014, 1.999999999999998224 ) ) ;
#3770=CARTESIAN_POINT ( 'NONE',  ( -3.845892476879857469, 6.661954734853424043, 13.99999999999999645 ) ) ;
#3772=CARTESIAN_POINT ( 'NONE',  ( 10.50003631213658117, 0.006025845833179007717, 14.00000000000000000 ) ) ;
#3777=CARTESIAN_POINT ( 'NONE',  ( -8.486979168634645632, -0.6954046021538184963, 1.999999999999998224 ) ) ;
#3778=CARTESIAN_POINT ( 'NONE',  ( 7.937472058415492526, 1.044590838406009858, 13.99999999999999645 ) ) ;
#3780=CARTESIAN_POINT ( 'NONE',  ( -5.391417556047953141, 8.653185861734563389, 14.00000000000000000 ) ) ;
#3785=CARTESIAN_POINT ( 'NONE',  ( -0.2403693791185868289, 7.265099133626555350, 14.00000000000000000 ) ) ;
#3786=CARTESIAN_POINT ( 'NONE',  ( 9.077580196901687160, 4.112174628513754371, 13.99999999999999645 ) ) ;
#3788=CARTESIAN_POINT ( 'NONE',  ( 3.247347166530789586, 6.590896817052466439, 14.00000000000000000 ) ) ;
#3790=CARTESIAN_POINT ( 'NONE',  ( -6.726831604608804582, -7.927219868180728213, 1.999999999999998224 ) ) ;
#3793=CARTESIAN_POINT ( 'NONE',  ( 5.499810765991186123, -5.314180015047517358, 1.999999999999998224 ) ) ;
#3795=CARTESIAN_POINT ( 'NONE',  ( -5.432680616552289621, 3.899654942172362748, 14.00000000000093792 ) ) ;
#3803=CARTESIAN_POINT ( 'NONE',  ( -7.080399483669990168, -6.208478756603781790, 1.999999999999998224 ) ) ;
#3805=CARTESIAN_POINT ( 'NONE',  ( 1.954797901281673633, -9.037865403626287986, 13.99999999999999645 ) ) ;
#3807=CARTESIAN_POINT ( 'NONE',  ( -2.331745755519268215, 9.978964459600446091, 14.00000000000000000 ) ) ;
#3813=CARTESIAN_POINT ( 'NONE',  ( 1.760389272475214373, -7.536528230137969686, 14.00000000000000000 ) ) ;
#3815=CARTESIAN_POINT ( 'NONE',  ( 7.631804465920718705, -6.689046765414282447, 13.99999999999999645 ) ) ;
#3818=CARTESIAN_POINT ( 'NONE',  ( 5.772253124442537242, -3.205917188173946997, 14.00000000000000000 ) ) ;
#3820=CARTESIAN_POINT ( 'NONE',  ( -7.044187934146015628, 6.598551529631267343, 1.999999999999998224 ) ) ;
#3823=CARTESIAN_POINT ( 'NONE',  ( -7.986673696634112751, -0.6581801297105769333, 1.999999999999998224 ) ) ;
#3825=ADVANCED_FACE ( 'NONE', ( #3832 ), #5244, .T. ) ;
#3827=CARTESIAN_POINT ( 'NONE',  ( -7.364573508975984062, 1.714675912027187943, 13.99999999999999645 ) ) ;
#3829=( NAMED_UNIT ( * ) PLANE_ANGLE_UNIT ( ) SI_UNIT ( $, .RADIAN. ) );
#3830=CARTESIAN_POINT ( 'NONE',  ( 4.853468040356245794, -8.397360160974407961, 1.999999999999998224 ) ) ;
#3832=FACE_OUTER_BOUND ( 'NONE', #3952, .T. ) ;
#3836=DIRECTION ( 'NONE',  ( -1.445602896647339163E-16, -0.000000000000000000, -1.000000000000000000 ) ) ;
#3838=CARTESIAN_POINT ( 'NONE',  ( -8.411612136543094920, -4.319922787977579226, 13.99999999999999645 ) ) ;
#3843=VERTEX_POINT ( 'NONE', #2160 ) ;
#3846=CARTESIAN_POINT ( 'NONE',  ( -6.742266116715659230, -1.811900715328871092, 14.00000000000000000 ) ) ;
#3847=CARTESIAN_POINT ( 'NONE',  ( -4.256527737015712631, -4.845957569453684499, 1.999999999999998224 ) ) ;
#3848=CARTESIAN_POINT ( 'NONE',  ( -6.334648143026945455, -2.872559841354017429, 14.00000000000000000 ) ) ;
#3850=CARTESIAN_POINT ( 'NONE',  ( 8.993528569561179964, -4.616306094804414784, 1.999999999999998224 ) ) ;
#3853=CARTESIAN_POINT ( 'NONE',  ( 3.247347166530788698, 6.590896817052186663, 1.999999999999998224 ) ) ;
#3854=CARTESIAN_POINT ( 'NONE',  ( 2.597146444261841491, -5.700021143261159828, 1.999999999999998224 ) ) ;
#3855=CARTESIAN_POINT ( 'NONE',  ( -0.8890388043606451962, 7.706404363472290520, 13.99999999999999645 ) ) ;
#3857=CARTESIAN_POINT ( 'NONE',  ( -9.692812185270616610, 2.758747493781260829, 1.999999999999998224 ) ) ;
#3863=CARTESIAN_POINT ( 'NONE',  ( 5.933674912743042817, -6.989438080420771193, 13.99999999999999645 ) ) ;
#3869=CARTESIAN_POINT ( 'NONE',  ( 3.208073253695060245, -8.107602109809697311, 14.00000000000000000 ) ) ;
#3870=CARTESIAN_POINT ( 'NONE',  ( -5.651290410005071152, 9.082320918485368821, 13.99999999999999645 ) ) ;
#3873=CARTESIAN_POINT ( 'NONE',  ( -5.416162817796315920, -4.301262981183149314, 14.00000000000000000 ) ) ;
#3875=CARTESIAN_POINT ( 'NONE',  ( 2.803319092186594030, 10.45862564946446760, 1.999999999999998224 ) ) ;
#3876=CARTESIAN_POINT ( 'NONE',  ( 2.869471237997715640, -6.613103333303074649, 13.99999999999999645 ) ) ;
#3878=CARTESIAN_POINT ( 'NONE',  ( 6.268835244667307904, -4.335177162149147279, 1.999999999999998224 ) ) ;
#3880=CARTESIAN_POINT ( 'NONE',  ( -6.505530684480628878, -3.618119970335913038, 13.99999999999999645 ) ) ;
#3882=( GEOMETRIC_REPRESENTATION_CONTEXT ( 3 ) GLOBAL_UNCERTAINTY_ASSIGNED_CONTEXT ( ( #2238 ) ) GLOBAL_UNIT_ASSIGNED_CONTEXT ( ( #397, #5349, #2701 ) ) REPRESENTATION_CONTEXT ( 'NONE', 'WORKASPACE' ) );
#3884=CARTESIAN_POINT ( 'NONE',  ( 2.667884741302309237, 9.975564253400264647, 1.999999999999998224 ) ) ;
#3890=CARTESIAN_POINT ( 'NONE',  ( 1.598519525623709692, 9.677660462521252782, 13.99999999999999645 ) ) ;
#3896=CARTESIAN_POINT ( 'NONE',  ( -3.987536574861253236, 7.161134007378101352, 14.00000000000000000 ) ) ;
#3897=CARTESIAN_POINT ( 'NONE',  ( -10.53467355220997526, 0.3418899515811328338, 13.99999999999999645 ) ) ;
#3899=PLANE ( 'NONE',  #5459 ) ;
#3900=CARTESIAN_POINT ( 'NONE',  ( -7.986673696634112751, -0.6581801297105769333, 14.00000000000000000 ) ) ;
#3905=CARTESIAN_POINT ( 'NONE',  ( 4.243312049792015372, -4.537448458213933833, 13.99999999999999645 ) ) ;
#3906=CARTESIAN_POINT ( 'NONE',  ( 3.857245400775495714, -7.804869966781508239, 1.999999999999998224 ) ) ;
#3907=PRODUCT_DEFINITION ( 'UNKNOWN', '', #2319, #2575 ) ;
#3910=CARTESIAN_POINT ( 'NONE',  ( 8.027649061863494140, -0.2602747315786821392, 1.999999999999998224 ) ) ;
#3911=CARTESIAN_POINT ( 'NONE',  ( 4.326322805050086373, -6.952463250691143237, 13.99999999999999645 ) ) ;
#3921=CARTESIAN_POINT ( 'NONE',  ( 8.396466517618241809, 3.163083589105052607, 13.99999999999999645 ) ) ;
#3928=CARTESIAN_POINT ( 'NONE',  ( -3.109042548464154621, -8.271822080921333864, 14.00000000000000000 ) ) ;
#3929=CARTESIAN_POINT ( 'NONE',  ( -9.381622446298930385, -4.629808687489260777, 13.99999999999999645 ) ) ;
#3933=CARTESIAN_POINT ( 'NONE',  ( -5.081985621531964981, 6.397721742171718518, 14.00000000000000000 ) ) ;
#3936=CARTESIAN_POINT ( 'NONE',  ( -0.7077576507783156501, 10.75210906117156995, 1.999999999999998224 ) ) ;
#3937=CARTESIAN_POINT ( 'NONE',  ( -4.310533329765174670, 5.077046166955135220, 13.99999999999952927 ) ) ;
#3938=CARTESIAN_POINT ( 'NONE',  ( 9.348788865897812883, 1.705571004836294646, 1.999999999999998224 ) ) ;
#3940=CARTESIAN_POINT ( 'NONE',  ( 7.025143070632193343, -0.1151745751371896220, 1.999999999999998224 ) ) ;
#3943=CARTESIAN_POINT ( 'NONE',  ( -5.183646570197097958, -3.010418922387011698, 1.999999999999998224 ) ) ;
#3946=CARTESIAN_POINT ( 'NONE',  ( 11.00000000000000355, -2.486888733138625796E-14, 7.999999999999996447 ) ) ;
#3948=CARTESIAN_POINT ( 'NONE',  ( -2.179108132477381332, -10.08557389312607278, 13.99999999999999645 ) ) ;
#3952=EDGE_LOOP ( 'NONE', ( #1700, #3632, #197, #3237 ) ) ;
#3954=CARTESIAN_POINT ( 'NONE',  ( 1.881113203117336319, 8.098457488330069509, 14.00000000000000000 ) ) ;
#3955=CARTESIAN_POINT ( 'NONE',  ( -6.576488680450179203, -0.2289623203888876135, 1.999999999999998224 ) ) ;
#3957=CARTESIAN_POINT ( 'NONE',  ( 6.037635170864974477, 5.848285684831325604, 14.00000000000000000 ) ) ;
#3959=CARTESIAN_POINT ( 'NONE',  ( -9.381622446299669349, -4.629808687489259889, 1.999999999999998224 ) ) ;
#3961=CARTESIAN_POINT ( 'NONE',  ( -0.5931392160223127874, -7.263020831007573896, 13.99999999999999645 ) ) ;
#3963=CARTESIAN_POINT ( 'NONE',  ( -1.515482495401827556, 9.129776367296644324, 1.999999999999998224 ) ) ;
#3964=CARTESIAN_POINT ( 'NONE',  ( 1.015216742983932274, 7.730330528320553896, 1.999999999999998224 ) ) ;
#3968=CARTESIAN_POINT ( 'NONE',  ( 5.460516619045266751, 3.400499599735594014, 1.999999999999998224 ) ) ;
#3972=CARTESIAN_POINT ( 'NONE',  ( 10.86297249782086105, 1.796588950249321304, 13.99999999999999645 ) ) ;
#3978=CARTESIAN_POINT ( 'NONE',  ( 5.612687125618119666, -6.603876269260188892, 14.00000000000000000 ) ) ;
#3979=CARTESIAN_POINT ( 'NONE',  ( 5.103689747953258582, 6.014827819656408892, 1.999999999999998224 ) ) ;
#3982=CARTESIAN_POINT ( 'NONE',  ( -1.001529162299639619, -8.740421795711004194, 14.00000000000000000 ) ) ;
#3985=CARTESIAN_POINT ( 'NONE',  ( 9.650319724628623419, 2.588775111615904567, 1.999999999999998224 ) ) ;
#3987=CARTESIAN_POINT ( 'NONE',  ( -4.892757975385434221, 9.527326283049751154, 1.999999999999998224 ) ) ;
#3988=CARTESIAN_POINT ( 'NONE',  ( -6.576488680450180979, -0.2289623203888878078, 13.99999999999999645 ) ) ;
#3990=CARTESIAN_POINT ( 'NONE',  ( 2.678407690932628871, -9.362678857629568085, 1.999999999999998224 ) ) ;
#3991=CARTESIAN_POINT ( 'NONE',  ( 7.812003909081975728, 1.689803927524521354, 1.999999999999998224 ) ) ;
#3996=CARTESIAN_POINT ( 'NONE',  ( 8.774740126074938473, 5.663528079765400847, 1.999999999999998224 ) ) ;
#4002=PLANE ( 'NONE',  #2640 ) ;
#4004=CARTESIAN_POINT ( 'NONE',  ( 3.605080641953931853, -9.570177220922108319, 13.99999999999999645 ) ) ;
#4009=CARTESIAN_POINT ( 'NONE',  ( -8.763921109941536614, 2.343993041296470903, 14.00000000000000000 ) ) ;
#4010=CARTESIAN_POINT ( 'NONE',  ( -2.919577271296705412, -6.733962781534540198, 1.999999999999998224 ) ) ;
#4013=CARTESIAN_POINT ( 'NONE',  ( -6.281085993838467552, -4.827840781182768382, 1.999999999999998224 ) ) ;
#4014=CARTESIAN_POINT ( 'NONE',  ( -3.109042548464154621, -8.271822080921333864, 14.00000000000000000 ) ) ;
#4017=CARTESIAN_POINT ( 'NONE',  ( -10.42442484909470046, -1.371544430045556373, 1.999999999999998224 ) ) ;
#4018=CARTESIAN_POINT ( 'NONE',  ( 5.733165789232424814, 2.946509839760390381, 14.00000000000000000 ) ) ;
#4019=CARTESIAN_POINT ( 'NONE',  ( -1.565980662507674648, 8.609317438862776228, 13.99999999999999645 ) ) ;
#4020=CARTESIAN_POINT ( 'NONE',  ( -0.1359230501496729582, -8.279147739301068398, 13.99999999999999645 ) ) ;
#4023=CARTESIAN_POINT ( 'NONE',  ( 5.059064342543293513, -7.053288479151686552, 1.999999999999998224 ) ) ;
#4024=CARTESIAN_POINT ( 'NONE',  ( 4.793600759081159346, 4.956424179878264447, 1.999999999999998224 ) ) ;
#4027=CARTESIAN_POINT ( 'NONE',  ( 11.00000000000000355, -2.486888733138625796E-14, 7.999999999999996447 ) ) ;
#4029=CARTESIAN_POINT ( 'NONE',  ( 9.602236826901936695, 4.172718697305983326, 1.999999999999998224 ) ) ;
#4030=CARTESIAN_POINT ( 'NONE',  ( -1.320393794063943416, 6.095439640211752774, 1.999999999999998224 ) ) ;
#4032=FACE_OUTER_BOUND ( 'NONE', #1124, .T. ) ;
#4034=EDGE_CURVE ( 'NONE', #3843, #2869, #2368, .T. ) ;
#4035=CARTESIAN_POINT ( 'NONE',  ( -9.381622446298930385, -4.629808687489260777, 13.99999999999999645 ) ) ;
#4040=CARTESIAN_POINT ( 'NONE',  ( -8.332455577112462208, 5.761155596212925722, 14.00000000000000000 ) ) ;
#4041=CARTESIAN_POINT ( 'NONE',  ( 7.132151089625187623, 3.519983721611797733, 1.999999999999998224 ) ) ;
#4042=CARTESIAN_POINT ( 'NONE',  ( -3.987536574860945038, 7.161134007378406885, 1.999999999999998224 ) ) ;
#4043=CARTESIAN_POINT ( 'NONE',  ( -8.547479018125100581, -2.754496926847988636, 14.00000000000000000 ) ) ;
#4045=CARTESIAN_POINT ( 'NONE',  ( 7.233280636258586860, 6.778630567624379211, 1.999999999999998224 ) ) ;
#4048=CARTESIAN_POINT ( 'NONE',  ( -8.486979168634645632, -0.6954046021538184963, 13.99999999999999645 ) ) ;
#4049=CARTESIAN_POINT ( 'NONE',  ( 3.471913601335457233, 7.039518430846527508, 13.99999999999999645 ) ) ;
#4050=CARTESIAN_POINT ( 'NONE',  ( 10.36702220812592223, 1.720931399333113676, 1.999999999999998224 ) ) ;
#4051=CARTESIAN_POINT ( 'NONE',  ( -2.263950162103713915, 8.438937471999857109, 1.999999999999998224 ) ) ;
#4052=( NAMED_UNIT ( * ) SI_UNIT ( $, .STERADIAN. ) SOLID_ANGLE_UNIT ( ) );
#4055=CARTESIAN_POINT ( 'NONE',  ( 6.496939485553420823, 0.4301729194711073623, 1.999999999999998224 ) ) ;
#4063=CARTESIAN_POINT ( 'NONE',  ( 5.099673838353210975, -8.834479793763010846, 13.99999999999999645 ) ) ;
#4066=EDGE_LOOP ( 'NONE', ( #1417, #3383, #3415, #865 ) ) ;
#4068=CARTESIAN_POINT ( 'NONE',  ( -9.445900372710701376, 3.550092993115766760, 14.00000000000000000 ) ) ;
#4069=CARTESIAN_POINT ( 'NONE',  ( -2.122668041763332347, 7.434468402752582250, 1.999999999999998224 ) ) ;
#4070=CARTESIAN_POINT ( 'NONE',  ( -8.913799778910963312, 1.613954699392611047, 1.999999999999998224 ) ) ;
#4071=CARTESIAN_POINT ( 'NONE',  ( -5.748891254250207083, -8.037420881458274380, 14.00000000000000000 ) ) ;
#4074=CARTESIAN_POINT ( 'NONE',  ( 0.1774200004017884857, 10.78715707688374614, 1.999999999999998224 ) ) ;
#4076=CARTESIAN_POINT ( 'NONE',  ( -6.681468852107525613, -5.130140014479350974, 13.99999999999999645 ) ) ;
#4077=CARTESIAN_POINT ( 'NONE',  ( 2.389076732465380548, -5.237771676862081449, 14.00000000000000000 ) ) ;
#4080=CARTESIAN_POINT ( 'NONE',  ( 7.024953159363688471, -4.052930060063556716, 1.999999999999998224 ) ) ;
#4084=CARTESIAN_POINT ( 'NONE',  ( -5.416162817796314144, -4.301262981183148426, 1.999999999999998224 ) ) ;
#4087=CARTESIAN_POINT ( 'NONE',  ( -4.184906021401388898, -5.457255036755482180, 1.999999999999998224 ) ) ;
#4092=VECTOR ( 'NONE', #3836, 1000.000000000000000 ) ;
#4099=CARTESIAN_POINT ( 'NONE',  ( -5.748891254250207083, -8.037420881458274380, 14.00000000000000000 ) ) ;
#4100=CARTESIAN_POINT ( 'NONE',  ( 5.862282306371745300, 6.688714470717011196, 1.999999999999998224 ) ) ;
#4102=CARTESIAN_POINT ( 'NONE',  ( 1.853537052132013363, -8.546502713975391075, 1.999999999999998224 ) ) ;
#4103=CARTESIAN_POINT ( 'NONE',  ( -8.290222237439158093, 3.747600907060152586, 14.00000000000000000 ) ) ;
#4105=CARTESIAN_POINT ( 'NONE',  ( 7.456063200420987691, 7.959410280423138140, 1.999999999999998224 ) ) ;
#4106=CARTESIAN_POINT ( 'NONE',  ( 1.730265954310492571, 6.073542049876724747, 14.00000000000000000 ) ) ;
#4107=CARTESIAN_POINT ( 'NONE',  ( -5.921118896519415919, 6.318058289644736369, 13.99999999999999645 ) ) ;
#4110=CARTESIAN_POINT ( 'NONE',  ( -3.139313036748680563, 9.741172307226465321, 1.999999999999998224 ) ) ;
#4113=CARTESIAN_POINT ( 'NONE',  ( 5.347643153870339283, -7.463670412152253242, 1.999999999999998224 ) ) ;
#4116=SHAPE_REPRESENTATION ( 'Spring Coil Unit', ( #1336 ), #2498 ) ;
#4117=CARTESIAN_POINT ( 'NONE',  ( -2.744490807750914030, 5.556819979548925481, 1.999999999999998224 ) ) ;
#4120=CARTESIAN_POINT ( 'NONE',  ( 6.004028658818956643, -2.715480180205985583, 1.999999999999998224 ) ) ;
#4124=CARTESIAN_POINT ( 'NONE',  ( 5.500000000000000000, 0.000000000000000000, 1.999999999999998224 ) ) ;
#4126=CARTESIAN_POINT ( 'NONE',  ( 11.00000000000000355, -2.488243985854232676E-14, 13.99999999999999645 ) ) ;
#4127=CARTESIAN_POINT ( 'NONE',  ( 2.678407690932720353, -9.362678857628843332, 14.00000000000000000 ) ) ;
#4128=CARTESIAN_POINT ( 'NONE',  ( 4.683456943470878819, 7.530568860026273015, 1.999999999999998224 ) ) ;
#4129=CARTESIAN_POINT ( 'NONE',  ( 8.477027301005913174, -1.108685663976167080, 1.999999999999998224 ) ) ;
#4130=CARTESIAN_POINT ( 'NONE',  ( -3.672794075660814617, 8.451992513476522362, 14.00000000000000000 ) ) ;
#4134=CARTESIAN_POINT ( 'NONE',  ( 2.227988792049260702, 5.923272706910787555, 14.00000000000000000 ) ) ;
#4135=CARTESIAN_POINT ( 'NONE',  ( -7.551678268146210016, 5.989845445213457964, 13.99999999999999645 ) ) ;
#4136=CARTESIAN_POINT ( 'NONE',  ( 9.925004466820084303, 3.374327561486830884, 1.999999999999998224 ) ) ;
#4138=CARTESIAN_POINT ( 'NONE',  ( -0.3010823416051299772, -9.281161307073867661, 1.999999999999998224 ) ) ;
#4141=CARTESIAN_POINT ( 'NONE',  ( 3.621982275015807051, -5.614208739972523787, 1.999999999999998224 ) ) ;
#4143=CARTESIAN_POINT ( 'NONE',  ( 7.526353627798827439, -0.2404185136226760222, 1.999999999999998224 ) ) ;
#4153=CARTESIAN_POINT ( 'NONE',  ( 5.933674912743041041, -6.989438080420770305, 1.999999999999998224 ) ) ;
#4155=CARTESIAN_POINT ( 'NONE',  ( -2.122668041763332347, 7.434468402752584026, 13.99999999999999645 ) ) ;
#4156=CARTESIAN_POINT ( 'NONE',  ( -5.391417556048331505, 8.653185861734561612, 1.999999999999998224 ) ) ;
#4161=ADVANCED_FACE ( 'NONE', ( #3115 ), #3399, .F. ) ;
#4162=CARTESIAN_POINT ( 'NONE',  ( 5.772253124442537242, -3.205917188173946997, 14.00000000000000000 ) ) ;
#4163=CARTESIAN_POINT ( 'NONE',  ( -9.533152408061619454, 0.1566715252476607312, 13.99999999999999645 ) ) ;
#4165=CARTESIAN_POINT ( 'NONE',  ( 5.500000000000001776, 0.000000000000000000, 14.00000000000000000 ) ) ;
#4168=CARTESIAN_POINT ( 'NONE',  ( -0.1462562576243746360, 8.775315755191545719, 1.999999999999998224 ) ) ;
#4171=CARTESIAN_POINT ( 'NONE',  ( -5.034899347481144538, -4.722558430572731503, 1.999999999999998224 ) ) ;
#4173=CARTESIAN_POINT ( 'NONE',  ( 4.064490656457592443, -6.524520197619557926, 1.999999999999998224 ) ) ;
#4177=B_SPLINE_SURFACE_WITH_KNOTS ( 'NONE', 1, 3, ( 
 ( #5437, #5062, #1492, #1471, #2824, #4576, #635, #2852, #1120, #200, #3627, #5386, #1444, #571, #2326, #2559, #3795, #773, #1582, #1612, #4207, #2994, #3370, #4288, #4319, #5552, #2526, #3341, #5125, #258, #4740, #2474, #2933, #3422, #1182, #343, #693, #5208, #4685, #4231, #4660, #368, #4710, #724, #1234, #4257, #2016, #5093, #806, #2961, #282, #745, #2497, #1266, #2097, #2126, #5607, #3880, #2039, #5635, #308, #2070, #3027, #3827, #5582, #1692, #5524, #1642, #3447, #2446, #3770, #3398, #1151, #3855, #2907, #5151, #1209, #5173, #1666, #4507, #102, #5342, #858, #2614, #4964, #3644, #4374, #1460, #1400, #3589, #4343, #394, #2155, #1887, #3161, #3911, #1727, #4908, #5427, #561, #5666, #1483, #4939, #1021, #2315, #537, #996, #4076, #76, #967, #504, #3216, #4048, #5240, #2725, #1917, #2342, #2261, #2779, #4107, #162, #3478, #1297, #4772, #4019, #1831, #129, #4477, #2287, #5401, #3053, #4797, #1858, #4534, #832, #3615, #5371, #1428, #3672, #3187, #2755, #590, #2584, #1547, #2894, #5542, #3302, #2841, #4594, #2491, #5022, #5051, #737, #1109, #1079, #2867, #4619, #678, #4647, #1598, #2432, #651, #2403, #4246, #4163, #1135, #5114, #217, #3329, #4135, #1972, #1048, #3358, #3726, #5485, #274, #4193, #714, #3240, #2055, #244, #2006, #1508, #2924, #1573, #3271, #3786, #3758, #4560, #1942, #1169, #5514, #5078, #2465, #4222, #3815, #2031, #4676, #297, #5570, #4988, #2810, #623, #2375, #189, #3696, #5453, #5255, #763, #359, #876, #3929, #5141, #4760, #2513, #3897, #5683, #3437, #2113, #416, #3041, #1287, #2574, #3870, #3413, #5165, #1741, #2174, #1226, #3496, #5622, #1682, #1200, #2949, #4702, #4360, #5194, #4277, #329, #1254, #2203, #4787 ),
 ( #1310, #4390, #2088, #2545, #3468, #3068, #4812, #2635, #3015, #445, #3847, #5598, #821, #3955, #1658, #846, #1630, #3389, #2979, #4728, #5654, #2602, #792, #4307, #4333, #382, #2143, #1713, #5229, #2281, #1419, #2334, #3180, #2717, #3608, #1764, #554, #5394, #4414, #3521, #5310, #3636, #1452, #2309, #14, #1371, #1015, #3153, #4930, #4874, #1794, #4527, #4010, #3583, #4469, #3210, #1825, #5336, #2773, #959, #3098, #931, #4500, #5281, #1338, #989, #581, #2749, #1394, #4846, #904, #4900, #4069, #528, #120, #2661, #1879, #468, #3550, #2226, #3979, #4958, #39, #4041, #96, #1851, #3126, #2685, #4440, #495, #2254, #67, #5363, #3233, #2801, #2023, #264, #4979, #5475, #5041, #236, #3348, #1476, #1909, #5445, #3666, #4213, #1159, #5420, #5013, #1994, #1127, #3777, #1589, #208, #5532, #1039, #4552, #1534, #5101, #613, #5506, #2914, #704, #4667, #729, #2421, #3749, #2365, #182, #4128, #4100, #3292, #153, #1499, #1934, #3689, #3262, #1961, #1071, #2833, #4584, #643, #2394, #2858, #4153, #3714, #1565, #4184, #1100, #4611, #3320, #670, #5068, #2883, #4638, #2454, #1620, #3803, #289, #2047, #1190, #2941, #5560, #4693, #3379, #5133, #2482, #4238, #5288, #4937, #2689, #3525, #4852, #4445, #2777, #3613, #3104, #4532, #2285, #2313, #5368, #3587, #4045, #1856, #3130, #502, #3985, #4505, #1398, #2667, #74, #4962, #5399, #45, #126, #1458, #3214, #1344, #908, #2207, #1800, #1375, #1426, #4879, #935, #3185, #4418, #472, #3557, #994, #3959, #2259, #5316, #4017, #1019, #1829, #5340, #3159, #4905, #965, #2753, #558, #2723, #4475, #535, #18, #100, #4074, #1885, #3642, #1770, #2231, #1505, #4105, #2891, #2373, #2839, #3327, #5020, #4191, #587 ) ),
 .UNSPECIFIED., .F., .F., .F.,
 ( 2, 2 ),
 ( 4, 2, 2, 2, 2, 2, 2, 2, 2, 2, 2, 2, 2, 2, 2, 2, 2, 2, 2, 2, 2, 2, 2, 2, 2, 2, 2, 2, 2, 2, 2, 2, 2, 2, 2, 2, 2, 2, 2, 2, 2, 2, 2, 2, 2, 2, 2, 2, 2, 2, 2, 2, 2, 2, 2, 2, 2, 2, 2, 2, 2, 2, 2, 2, 2, 2, 2, 2, 2, 2, 2, 2, 2, 2, 2, 2, 2, 2, 2, 2, 2, 2, 2, 2, 2, 2, 2, 2, 2, 2, 2, 2, 2, 2, 2, 2, 2, 2, 2, 2, 2, 2, 2, 2, 2, 2, 2, 2, 2, 2, 2, 2, 2, 2, 2, 2, 2, 2, 2, 2, 4 ),
 ( 0.000000000000000000, 0.4799999999999999822 ),
 ( 0.000000000000000000, 0.01562500000000000000, 0.03125000000000000000, 0.04687500000000000000, 0.06250000000000000000, 0.07812500000000000000, 0.09375000000000000000, 0.1093750000000000000, 0.1250000000000000000, 0.1328125000000000000, 0.1406250000000000000, 0.1484375000000000000, 0.1562500000000000000, 0.1640625000000000000, 0.1718750000000000000, 0.1796875000000000000, 0.1875000000000000000, 0.1953125000000000000, 0.2031250000000000000, 0.2109375000000000000, 0.2187500000000000000, 0.2265625000000000000, 0.2343750000000000000, 0.2421875000000000000, 0.2500000000000000000, 0.2578125000000000000, 0.2656250000000000000, 0.2734375000000000000, 0.2812500000000000000, 0.2890625000000000000, 0.2968750000000000000, 0.3046875000000000000, 0.3125000000000000000, 0.3203125000000000000, 0.3281250000000000000, 0.3359375000000000000, 0.3437500000000000000, 0.3515625000000000000, 0.3593750000000000000, 0.3671875000000000000, 0.3750000000000000000, 0.3828125000000000000, 0.3906250000000000000, 0.3984375000000000000, 0.4062500000000000000, 0.4140625000000000000, 0.4218750000000000000, 0.4296875000000000000, 0.4375000000000000000, 0.4453125000000000000, 0.4531250000000000000, 0.4609375000000000000, 0.4687500000000000000, 0.4765625000000000000, 0.4843750000000000000, 0.4921875000000000000, 0.5000000000000000000, 0.5078125000000000000, 0.5156250000000000000, 0.5234375000000000000, 0.5312500000000000000, 0.5390625000000000000, 0.5468750000000000000, 0.5546875000000000000, 0.5625000000000000000, 0.5703125000000000000, 0.5781250000000000000, 0.5859375000000000000, 0.5937500000000000000, 0.6015625000000000000, 0.6093750000000000000, 0.6171875000000000000, 0.6250000000000000000, 0.6328125000000000000, 0.6406250000000000000, 0.6484375000000000000, 0.6562500000000000000, 0.6640625000000000000, 0.6718750000000000000, 0.6796875000000000000, 0.6875000000000000000, 0.6953125000000000000, 0.7031250000000000000, 0.7109375000000000000, 0.7187500000000000000, 0.7265625000000000000, 0.7343750000000000000, 0.7421875000000000000, 0.7500000000000000000, 0.7578125000000000000, 0.7656250000000000000, 0.7734375000000000000, 0.7812500000000000000, 0.7890625000000000000, 0.7968750000000000000, 0.8046875000000000000, 0.8125000000000000000, 0.8203125000000000000, 0.8281250000000000000, 0.8359375000000000000, 0.8437500000000000000, 0.8515625000000000000, 0.8593750000000000000, 0.8671875000000000000, 0.8750000000000000000, 0.8828125000000000000, 0.8906250000000000000, 0.8984375000000000000, 0.9062500000000000000, 0.9140625000000000000, 0.9218750000000000000, 0.9296875000000000000, 0.9375000000000000000, 0.9453125000000000000, 0.9531250000000000000, 0.9609375000000000000, 0.9687500000000000000, 0.9765625000000000000, 0.9843750000000000000, 0.9921875000000000000, 1.000000000000000000 ),
 .UNSPECIFIED. ) ;
#4184=CARTESIAN_POINT ( 'NONE',  ( 3.388254439433305176, -8.575817650944026482, 1.999999999999998224 ) ) ;
#4185=CARTESIAN_POINT ( 'NONE',  ( -3.441860715206332522, -7.602597312514155270, 13.99999999999999645 ) ) ;
#4186=CARTESIAN_POINT ( 'NONE',  ( 8.269507991092027055, 6.356934974246627235, 14.00000000000000000 ) ) ;
#4191=CARTESIAN_POINT ( 'NONE',  ( 10.98697916625148707, 0.8999353979983775176, 1.999999999999998224 ) ) ;
#4192=CARTESIAN_POINT ( 'NONE',  ( -1.987635485262058577, 6.951293809708866789, 14.00000000000000000 ) ) ;
#4193=CARTESIAN_POINT ( 'NONE',  ( -0.7976699882156008670, 9.736979168371714621, 13.99999999999999645 ) ) ;
#4196=CARTESIAN_POINT ( 'NONE',  ( 4.062840028443491569, -5.287223670286397059, 14.00000000000000000 ) ) ;
#4199=CARTESIAN_POINT ( 'NONE',  ( -10.53467355221071777, 0.3418899515810866485, 1.999999999999998224 ) ) ;
#4202=CARTESIAN_POINT ( 'NONE',  ( 1.540339863274624577, 7.144097608501353669, 1.999999999999998224 ) ) ;
#4204=CARTESIAN_POINT ( 'NONE',  ( -6.065725208710914806, -3.376743199310592747, 1.999999999999998224 ) ) ;
#4207=CARTESIAN_POINT ( 'NONE',  ( -2.466819000628047487, 6.242838961510106977, 13.99999999999999645 ) ) ;
#4213=CARTESIAN_POINT ( 'NONE',  ( -5.741039858921414663, -6.128965587877393872, 1.999999999999998224 ) ) ;
#4215=CARTESIAN_POINT ( 'NONE',  ( 5.857810772706378621, -5.665644577056677456, 13.99999999999999645 ) ) ;
#4217=ORIENTED_EDGE ( 'NONE', *, *, #2485, .F. ) ;
#4221=CARTESIAN_POINT ( 'NONE',  ( -2.547213823411295319, 6.752160688201485961, 14.00000000000000000 ) ) ;
#4222=CARTESIAN_POINT ( 'NONE',  ( 8.595497693524210447, -5.345940745659388149, 13.99999999999999645 ) ) ;
#4223=CARTESIAN_POINT ( 'NONE',  ( 6.160418207306094018, 1.983851483784787373, 14.00000000000000000 ) ) ;
#4226=CARTESIAN_POINT ( 'NONE',  ( 9.599547022228483328, -3.085197981542975310, 1.999999999999998224 ) ) ;
#4229=CARTESIAN_POINT ( 'NONE',  ( 5.053476174607396842, -5.757900651972986950, 1.999999999999998224 ) ) ;
#4231=CARTESIAN_POINT ( 'NONE',  ( 6.460119401626726265, -2.924461030940389783, 13.99999999999999645 ) ) ;
#4238=CARTESIAN_POINT ( 'NONE',  ( -8.402144917908874078, 4.670158400850170644, 1.999999999999998224 ) ) ;
#4239=CARTESIAN_POINT ( 'NONE',  ( 6.019515613300196577, 7.843576796802396167, 13.99999999999999645 ) ) ;
#4240=CARTESIAN_POINT ( 'NONE',  ( -4.668631340267771712, 9.078485505802326827, 14.00000000000000000 ) ) ;
#4245=CARTESIAN_POINT ( 'NONE',  ( 1.540339863274486465, 7.144097608501355445, 14.00000000000000000 ) ) ;
#4246=CARTESIAN_POINT ( 'NONE',  ( -9.500632974893353122, -0.6255030753161997525, 13.99999999999999645 ) ) ;
#4248=CARTESIAN_POINT ( 'NONE',  ( 7.320916985966520407, 1.587212364775818285, 14.00000000000000000 ) ) ;
#4250=CARTESIAN_POINT ( 'NONE',  ( 2.810994617404584783, -9.846529629019117991, 1.999999999999998224 ) ) ;
#4254=CARTESIAN_POINT ( 'NONE',  ( -5.081985621532272290, 6.397721742171409431, 1.999999999999998224 ) ) ;
#4257=CARTESIAN_POINT ( 'NONE',  ( 2.869471237997715640, -6.613103333303074649, 13.99999999999999645 ) ) ;
#4260=CARTESIAN_POINT ( 'NONE',  ( -10.03347820201762630, 0.3196629254998830660, 1.999999999999998224 ) ) ;
#4268=CARTESIAN_POINT ( 'NONE',  ( 4.683456943470878819, 7.530568860026274791, 13.99999999999999645 ) ) ;
#4276=CARTESIAN_POINT ( 'NONE',  ( 2.161943361801395014, -6.363123982928430067, 14.00000000000000000 ) ) ;
#4277=CARTESIAN_POINT ( 'NONE',  ( 10.06493078320225010, 4.366638945734137245, 13.99999999999999645 ) ) ;
#4280=CARTESIAN_POINT ( 'NONE',  ( 1.103627080440590547, -6.655442145117441477, 14.00000000000000000 ) ) ;
#4282=CARTESIAN_POINT ( 'NONE',  ( -5.250997584835956467, 8.145342823910020513, 1.999999999999998224 ) ) ;
#4285=CARTESIAN_POINT ( 'NONE',  ( 5.528193227148988420, 6.314447692498917242, 1.999999999999998224 ) ) ;
#4288=CARTESIAN_POINT ( 'NONE',  ( 0.2194671214740386012, 6.774136816532214667, 13.99999999999999645 ) ) ;
#4291=CARTESIAN_POINT ( 'NONE',  ( -7.559400777704422758, -6.425066744314571920, 1.999999999999998224 ) ) ;
#4299=CARTESIAN_POINT ( 'NONE',  ( -4.679820741050984445, -8.111215689329295486, 13.99999999999999645 ) ) ;
#4302=LINE ( 'NONE', #3009, #3272 ) ;
#4306=CARTESIAN_POINT ( 'NONE',  ( -4.895455514773497718, -6.178604150901620073, 14.00000000000000000 ) ) ;
#4307=CARTESIAN_POINT ( 'NONE',  ( 0.2194671214740537279, 6.774136816532212890, 1.999999999999998224 ) ) ;
#4310=CARTESIAN_POINT ( 'NONE',  ( -2.547213823411295319, 6.752160688201485961, 14.00000000000000000 ) ) ;
#4313=CARTESIAN_POINT ( 'NONE',  ( -9.406456921418630657, 1.708717176649225511, 1.999999999999998224 ) ) ;
#4315=CARTESIAN_POINT ( 'NONE',  ( 5.586635445632386343, -4.430858740432560339, 13.99999999999999645 ) ) ;
#4317=CARTESIAN_POINT ( 'NONE',  ( -2.020383375745208987, -7.552201994671270846, 1.999999999999998224 ) ) ;
#4319=CARTESIAN_POINT ( 'NONE',  ( 0.7762864403411009473, 6.746413643992396736, 13.99999999999999645 ) ) ;
#4320=CARTESIAN_POINT ( 'NONE',  ( 4.264126983937991611, 9.433107915010285893, 1.999999999999998224 ) ) ;
#4326=CARTESIAN_POINT ( 'NONE',  ( -5.893815055328263774, 7.676334994785688259, 13.99999999999999645 ) ) ;
#4332=CARTESIAN_POINT ( 'NONE',  ( 1.147089839255721166, -8.682979827542890661, 14.00000000000000000 ) ) ;
#4333=CARTESIAN_POINT ( 'NONE',  ( 0.7762864403411611214, 6.746413643992394960, 1.999999999999998224 ) ) ;
#4335=CARTESIAN_POINT ( 'NONE',  ( 6.929006764466010715, 4.804313515625074693, 14.00000000000000000 ) ) ;
#4337=CARTESIAN_POINT ( 'NONE',  ( 9.199536834907135585, 5.930433524309127513, 1.999999999999998224 ) ) ;
#4339=CARTESIAN_POINT ( 'NONE',  ( 0.7762864403411009473, 6.746413643992396736, 13.99999999999999645 ) ) ;
#4341=CARTESIAN_POINT ( 'NONE',  ( -7.588772809867561087, -4.728083520432016407, 1.999999999999998224 ) ) ;
#4342=CARTESIAN_POINT ( 'NONE',  ( -7.211577653563208123, 2.317451195016654530, 1.999999999999998224 ) ) ;
#4343=CARTESIAN_POINT ( 'NONE',  ( 7.565999024956893138, -2.848076369834590338, 13.99999999999999645 ) ) ;
#4346=CARTESIAN_POINT ( 'NONE',  ( -6.398096652174580790, -7.548242073784104278, 1.999999999999998224 ) ) ;
#4352=CARTESIAN_POINT ( 'NONE',  ( 4.043470907200354070, 7.877814422642792636, 13.99999999999999645 ) ) ;
#4359=CARTESIAN_POINT ( 'NONE',  ( 2.543939756934300966, 7.929199913827024382, 14.00000000000000000 ) ) ;
#4360=CARTESIAN_POINT ( 'NONE',  ( 8.671201137382265500, 6.657490096169393468, 13.99999999999999645 ) ) ;
#4363=CARTESIAN_POINT ( 'NONE',  ( 8.370269057508139099, -1.803949267857856142, 14.00000000000000000 ) ) ;
#4369=CARTESIAN_POINT ( 'NONE',  ( -7.375360291558942905, -1.341686286798741357, 13.99999999999999645 ) ) ;
#4371=CARTESIAN_POINT ( 'NONE',  ( 9.522148329495122354, -0.6196525284525815636, 1.999999999999998224 ) ) ;
#4373=CARTESIAN_POINT ( 'NONE',  ( -4.492165532403227246, -5.853844512260856447, 1.999999999999998224 ) ) ;
#4374=CARTESIAN_POINT ( 'NONE',  ( 7.937472058415492526, 1.044590838406009858, 13.99999999999999645 ) ) ;
#4377=CARTESIAN_POINT ( 'NONE',  ( -1.336592501075286599, -5.709464570123371274, 1.999999999999998224 ) ) ;
#4381=CARTESIAN_POINT ( 'NONE',  ( 11.00000000000000355, -2.485533480423018915E-14, 1.999999999999998224 ) ) ;
#4382=CARTESIAN_POINT ( 'NONE',  ( -0.7077576507784110182, 10.75210906117156995, 13.99999999999999645 ) ) ;
#4389=CARTESIAN_POINT ( 'NONE',  ( -6.185289998984974780, -6.402116997106622520, 14.00000000000000000 ) ) ;
#4390=CARTESIAN_POINT ( 'NONE',  ( 6.026041665150464688, -0.9817477132364114123, 1.999999999999998224 ) ) ;
#4392=CARTESIAN_POINT ( 'NONE',  ( -7.945923533235638381, 1.308497053349305883, 14.00000000000000000 ) ) ;
#4395=CARTESIAN_POINT ( 'NONE',  ( 10.06493078320224832, 4.366638945733749111, 1.999999999999998224 ) ) ;
#4396=CARTESIAN_POINT ( 'NONE',  ( 3.909482108038855319, 5.648312977191786821, 13.99999999999999645 ) ) ;
#4397=PRODUCT_CONTEXT ( 'NONE', #2768, 'mechanical' ) ;
#4398=CARTESIAN_POINT ( 'NONE',  ( 9.123540010895986541, -2.926742269086382908, 1.999999999999998224 ) ) ;
#4399=CARTESIAN_POINT ( 'NONE',  ( 5.194219494279652238, 4.554949839096303243, 1.999999999999998224 ) ) ;
#4402=CARTESIAN_POINT ( 'NONE',  ( 2.227988792049259814, 5.923272706911028251, 1.999999999999998224 ) ) ;
#4405=CARTESIAN_POINT ( 'NONE',  ( 5.500000000000000000, 0.000000000000000000, 1.999999999999998224 ) ) ;
#4408=DIRECTION ( 'NONE',  ( -1.000000000000000000, 0.000000000000000000, 0.000000000000000000 ) ) ;
#4412=CARTESIAN_POINT ( 'NONE',  ( 7.716263785693138644, -3.801003699433110228, 14.00000000000000000 ) ) ;
#4414=CARTESIAN_POINT ( 'NONE',  ( 6.824478893064961582, -1.828844244265459329, 1.999999999999998224 ) ) ;
#4416=CARTESIAN_POINT ( 'NONE',  ( -0.1241967792452473573, -7.777596356722547455, 14.00000000000000000 ) ) ;
#4417=ORIENTED_EDGE ( 'NONE', *, *, #5526, .T. ) ;
#4418=CARTESIAN_POINT ( 'NONE',  ( -6.045729098460860484, -8.441868823237593134, 1.999999999999998224 ) ) ;
#4421=CARTESIAN_POINT ( 'NONE',  ( 4.793600759081160234, 4.956424179878266223, 13.99999999999999645 ) ) ;
#4423=CARTESIAN_POINT ( 'NONE',  ( 4.853468040356245794, -8.397360160974407961, 1.999999999999998224 ) ) ;
#4424=CARTESIAN_POINT ( 'NONE',  ( 6.997680802075242568, 0.4609939245310665235, 1.999999999999998224 ) ) ;
#4427=CARTESIAN_POINT ( 'NONE',  ( 3.896371052708264227, -4.167854722424304548, 1.999999999999998224 ) ) ;
#4428=CARTESIAN_POINT ( 'NONE',  ( 6.315449825284093599, 1.474116854620456163, 1.999999999999998224 ) ) ;
#4439=CARTESIAN_POINT ( 'NONE',  ( 0.3244988297792451570, -9.772062696132405080, 14.00000000000000000 ) ) ;
#4440=CARTESIAN_POINT ( 'NONE',  ( 7.992346231215205599, -0.9198489573344823533, 1.999999999999998224 ) ) ;
#4441=CARTESIAN_POINT ( 'NONE',  ( -5.395431796987671724, -5.765308706272893602, 1.999999999999998224 ) ) ;
#4442=ADVANCED_FACE ( 'NONE', ( #4752 ), #376, .T. ) ;
#4443=CARTESIAN_POINT ( 'NONE',  ( -7.652305818843811558, 2.590529227167490234, 14.00000000000000000 ) ) ;
#4445=CARTESIAN_POINT ( 'NONE',  ( -3.127066335681005338, 9.214240776399423183, 1.999999999999998224 ) ) ;
#4448=CARTESIAN_POINT ( 'NONE',  ( -5.210352092881700869, -6.569156856910654874, 13.99999999999999645 ) ) ;
#4450=CARTESIAN_POINT ( 'NONE',  ( -8.763921109942213405, 2.343993041296470459, 1.999999999999998224 ) ) ;
#4451=CARTESIAN_POINT ( 'NONE',  ( 3.471913601335177013, 7.039518430846525732, 1.999999999999998224 ) ) ;
#4455=CARTESIAN_POINT ( 'NONE',  ( 10.50003631213657762, 0.006025845833179020727, 1.999999999999998224 ) ) ;
#4457=CARTESIAN_POINT ( 'NONE',  ( -3.987231204391976203, 4.693390172671164429, 1.999999999999412914 ) ) ;
#4462=CARTESIAN_POINT ( 'NONE',  ( -6.726831604608805470, -7.927219868181097695, 13.99999999999999645 ) ) ;
#4468=CARTESIAN_POINT ( 'NONE',  ( -9.692812185271368008, 2.758747493781260385, 14.00000000000000000 ) ) ;
#4469=CARTESIAN_POINT ( 'NONE',  ( -4.492165532403227246, -5.853844512260856447, 1.999999999999998224 ) ) ;
#4471=CARTESIAN_POINT ( 'NONE',  ( -1.001529162299556797, -8.740421795711002417, 1.999999999999998224 ) ) ;
#4472=CARTESIAN_POINT ( 'NONE',  ( -3.609299841826104416, -9.156952235374472338, 14.00000000000000000 ) ) ;
#4475=CARTESIAN_POINT ( 'NONE',  ( -4.892757975385434221, 9.527326283049751154, 1.999999999999998224 ) ) ;
#4476=CARTESIAN_POINT ( 'NONE',  ( 5.526041665711820983, -0.8982374663919268087, 14.00000000000000000 ) ) ;
#4477=CARTESIAN_POINT ( 'NONE',  ( 1.999247522871012483, 8.586038698135613600, 13.99999999999999645 ) ) ;
#4478=CARTESIAN_POINT ( 'NONE',  ( 5.381714297850043849, -6.137309488907495947, 13.99999999999999645 ) ) ;
#4481=CARTESIAN_POINT ( 'NONE',  ( -3.110890340275590304, -5.031137978950551037, 14.00000000000000000 ) ) ;
#4483=CARTESIAN_POINT ( 'NONE',  ( 2.519353604429720228, -7.832629354751149187, 1.999999999999998224 ) ) ;
#4487=CARTESIAN_POINT ( 'NONE',  ( 8.269507991092025279, 6.356934974247397285, 1.999999999999998224 ) ) ;
#4494=CARTESIAN_POINT ( 'NONE',  ( -1.342170334697156742, -10.21728332006373030, 13.99999999999999645 ) ) ;
#4499=CARTESIAN_POINT ( 'NONE',  ( -2.067895747887562141, -9.596367745172036834, 14.00000000000000000 ) ) ;
#4500=CARTESIAN_POINT ( 'NONE',  ( -7.519441789400336695, 0.4931591957933217363, 1.999999999999998224 ) ) ;
#4502=CARTESIAN_POINT ( 'NONE',  ( -8.757712506721389900, -2.046213373001789737, 1.999999999999998224 ) ) ;
#4503=CARTESIAN_POINT ( 'NONE',  ( 3.433597602020987072, -9.098706718024024198, 14.00000000000000000 ) ) ;
#4505=CARTESIAN_POINT ( 'NONE',  ( 9.843274586260609027, 1.790275038161348364, 1.999999999999998224 ) ) ;
#4507=CARTESIAN_POINT ( 'NONE',  ( 4.585040342817689130, 6.402697129001494680, 13.99999999999999645 ) ) ;
#4510=CARTESIAN_POINT ( 'NONE',  ( -6.708753103182418798, 7.642576097240645794, 1.999999999999998224 ) ) ;
#4511=ORIENTED_EDGE ( 'NONE', *, *, #1888, .F. ) ;
#4512=CARTESIAN_POINT ( 'NONE',  ( 8.164254108709977586, -4.026826083952141033, 1.999999999999998224 ) ) ;
#4515=CARTESIAN_POINT ( 'NONE',  ( -2.717942380035140104, -6.274577315194988181, 1.999999999999998224 ) ) ;
#4517=CARTESIAN_POINT ( 'NONE',  ( -6.734745854535898246, 2.161492950161982396, 1.999999999999998224 ) ) ;
#4526=CARTESIAN_POINT ( 'NONE',  ( 9.527640065891670673, 0.1642265212908743666, 14.00000000000000000 ) ) ;
#4527=CARTESIAN_POINT ( 'NONE',  ( -2.352725117874390204, -6.938351456669183293, 1.999999999999998224 ) ) ;
#4528=CARTESIAN_POINT ( 'NONE',  ( -7.963215149404742732, -4.094909132697305054, 1.999999999999998224 ) ) ;
#4530=CARTESIAN_POINT ( 'NONE',  ( -10.03347820201837237, 0.3196629254998830660, 14.00000000000000000 ) ) ;
#4532=CARTESIAN_POINT ( 'NONE',  ( 1.598519525623709248, 9.677660462521251006, 1.999999999999998224 ) ) ;
#4533=CARTESIAN_POINT ( 'NONE',  ( 4.513069810084764377, -3.445129632735343339, 14.00000000000000000 ) ) ;
#4534=CARTESIAN_POINT ( 'NONE',  ( 7.344045208303976224, 5.086154276871550195, 13.99999999999999645 ) ) ;
#4535=CARTESIAN_POINT ( 'NONE',  ( -8.929154442179981999, -4.413097966322209409, 1.999999999999998224 ) ) ;
#4538=CARTESIAN_POINT ( 'NONE',  ( -8.440272934376206848, 1.393994921405934173, 1.999999999999998224 ) ) ;
#4541=CARTESIAN_POINT ( 'NONE',  ( -6.041022033915842471, 3.753782041846908779, 1.999999999999998224 ) ) ;
#4543=CARTESIAN_POINT ( 'NONE',  ( 6.941605245898607279, 2.746080019686067519, 1.999999999999998224 ) ) ;
#4551=CARTESIAN_POINT ( 'NONE',  ( -7.966005157978615969, 4.422220743486623640, 14.00000000000000000 ) ) ;
#4552=CARTESIAN_POINT ( 'NONE',  ( -7.245889760505162869, 4.668767092638087313, 1.999999999999998224 ) ) ;
#4554=CARTESIAN_POINT ( 'NONE',  ( -5.081985621532272290, 6.397721742171409431, 1.999999999999998224 ) ) ;
#4555=CARTESIAN_POINT ( 'NONE',  ( -8.929154442179243034, -4.413097966322579779, 14.00000000000000000 ) ) ;
#4559=CARTESIAN_POINT ( 'NONE',  ( -3.110890340275590304, -5.031137978950551037, 14.00000000000000000 ) ) ;
#4560=CARTESIAN_POINT ( 'NONE',  ( 9.843274586260610803, 1.790275038161259991, 13.99999999999999645 ) ) ;
#4562=CARTESIAN_POINT ( 'NONE',  ( -3.609299841826103972, -9.156952235374472338, 1.999999999999998224 ) ) ;
#4566=CARTESIAN_POINT ( 'NONE',  ( -1.565980662507674426, 8.609317438863394401, 1.999999999999998224 ) ) ;
#4570=CARTESIAN_POINT ( 'NONE',  ( 4.443413384189978110, 4.597174039215664365, 1.999999999999998224 ) ) ;
#4573=CARTESIAN_POINT ( 'NONE',  ( -1.987635485262058133, 6.951293809708865012, 1.999999999999998224 ) ) ;
#4576=CARTESIAN_POINT ( 'NONE',  ( 2.597146444261842824, -5.700021143261160717, 13.99999999999999645 ) ) ;
#4584=CARTESIAN_POINT ( 'NONE',  ( 8.454926800554316557, -3.338224220245900042, 1.999999999999998224 ) ) ;
#4586=CARTESIAN_POINT ( 'NONE',  ( -8.126042061586270293, 2.755650963504471473, 13.99999999999999645 ) ) ;
#4587=CARTESIAN_POINT ( 'NONE',  ( 8.618507686538960044, 3.909830026711944573, 1.999999999999998224 ) ) ;
#4588=CARTESIAN_POINT ( 'NONE',  ( -5.592500163774714039, 7.275211197852027745, 14.00000000000000000 ) ) ;
#4593=CARTESIAN_POINT ( 'NONE',  ( 6.445330636073146380, -1.168293168414177741, 14.00000000000000000 ) ) ;
#4594=CARTESIAN_POINT ( 'NONE',  ( 3.388254439433305176, -8.575817650944683734, 13.99999999999999645 ) ) ;
#4595=CARTESIAN_POINT ( 'NONE',  ( -5.391417556048331505, 8.653185861734561612, 1.999999999999998224 ) ) ;
#4597=CARTESIAN_POINT ( 'NONE',  ( 2.701324588234195190, 8.405562337868014211, 1.999999999999998224 ) ) ;
#4600=CARTESIAN_POINT ( 'NONE',  ( 1.103627080440590102, -6.655442145117440589, 1.999999999999998224 ) ) ;
#4602=CARTESIAN_POINT ( 'NONE',  ( 6.340368144647110071, -1.697206311170896598, 1.999999999999998224 ) ) ;
#4610=CARTESIAN_POINT ( 'NONE',  ( 7.108868828250529681, 7.597268273415099138, 14.00000000000000000 ) ) ;
#4611=CARTESIAN_POINT ( 'NONE',  ( 1.208067634251008604, -9.180948453718620783, 1.999999999999998224 ) ) ;
#4612=CARTESIAN_POINT ( 'NONE',  ( -7.245889760505164645, 4.668767092638694827, 13.99999999999999645 ) ) ;
#4618=CARTESIAN_POINT ( 'NONE',  ( 5.499810765991187012, -5.314180015047230476, 14.00000000000000000 ) ) ;
#4619=CARTESIAN_POINT ( 'NONE',  ( -5.337360893036674270, -7.710592058383929803, 13.99999999999999645 ) ) ;
#4621=CARTESIAN_POINT ( 'NONE',  ( 6.496939485553422600, 0.4301729194711386151, 14.00000000000000000 ) ) ;
#4623=CARTESIAN_POINT ( 'NONE',  ( -3.798941939731882655, -9.621416145858376012, 1.999999999999998224 ) ) ;
#4626=CARTESIAN_POINT ( 'NONE',  ( 2.672042568001582019, -6.151894458593051063, 1.999999999999998224 ) ) ;
#4628=CARTESIAN_POINT ( 'NONE',  ( -5.370374743918785221, 4.702532619530842339, 1.999999999999998224 ) ) ;
#4638=CARTESIAN_POINT ( 'NONE',  ( -4.679820741051314847, -8.111215689328634681, 1.999999999999998224 ) ) ;
#4640=ADVANCED_FACE ( 'NONE', ( #2116 ), #3899, .T. ) ;
#4641=CARTESIAN_POINT ( 'NONE',  ( -3.845892476879857469, 6.661954734853424043, 13.99999999999999645 ) ) ;
#4646=CARTESIAN_POINT ( 'NONE',  ( -4.089163901200158158, 5.898691170884823975, 14.00000000000000000 ) ) ;
#4647=CARTESIAN_POINT ( 'NONE',  ( -7.080399483669658878, -6.208478756603783566, 13.99999999999999645 ) ) ;
#4649=CARTESIAN_POINT ( 'NONE',  ( -0.2403693791185868289, 7.265099133626555350, 14.00000000000000000 ) ) ;
#4652=CARTESIAN_POINT ( 'NONE',  ( -9.247243397276459831, 2.478494142799053446, 1.999999999999998224 ) ) ;
#4656=CARTESIAN_POINT ( 'NONE',  ( -1.390902631672706002, -7.679604985168658970, 1.999999999999998224 ) ) ;
#4658=CARTESIAN_POINT ( 'NONE',  ( -0.1241967792452471353, -7.777596356722545679, 1.999999999999998224 ) ) ;
#4660=CARTESIAN_POINT ( 'NONE',  ( 6.209839678909983895, -3.451293940533043614, 13.99999999999999645 ) ) ;
#4667=CARTESIAN_POINT ( 'NONE',  ( -1.565980662507674426, 8.609317438863394401, 1.999999999999998224 ) ) ;
#4669=CARTESIAN_POINT ( 'NONE',  ( 8.164254108709979363, -4.026826083952141921, 13.99999999999999645 ) ) ;
#4672=CARTESIAN_POINT ( 'NONE',  ( 10.50003631213657407, 0.006025845833178966951, 1.999999999999998668 ) ) ;
#4675=CARTESIAN_POINT ( 'NONE',  ( 4.064490656458173312, -6.524520197619847472, 14.00000000000000000 ) ) ;
#4676=CARTESIAN_POINT ( 'NONE',  ( 5.800093669798302543, -8.375184749302979625, 13.99999999999999645 ) ) ;
#4677=CARTESIAN_POINT ( 'NONE',  ( 6.941605245898609056, 2.746080019685927187, 14.00000000000000000 ) ) ;
#4679=CARTESIAN_POINT ( 'NONE',  ( 9.843274586260609027, 1.790275038161348364, 1.999999999999998224 ) ) ;
#4683=CARTESIAN_POINT ( 'NONE',  ( -7.301858691287086423, -3.172613069824385068, 1.999999999999998224 ) ) ;
#4685=CARTESIAN_POINT ( 'NONE',  ( 6.824478893064963358, -1.828844244265460217, 13.99999999999999645 ) ) ;
#4687=CARTESIAN_POINT ( 'NONE',  ( -9.273719170356997665, -3.669762015052091098, 1.999999999999998224 ) ) ;
#4693=CARTESIAN_POINT ( 'NONE',  ( -9.533152408061617678, 0.1566715252477025866, 1.999999999999998224 ) ) ;
#4694=CARTESIAN_POINT ( 'NONE',  ( 5.862282306371745300, 6.688714470717012972, 13.99999999999999645 ) ) ;
#4701=CARTESIAN_POINT ( 'NONE',  ( 2.369394374793903246, -7.353877281245580377, 14.00000000000000000 ) ) ;
#4702=CARTESIAN_POINT ( 'NONE',  ( 7.456063200421762183, 7.959410280422752670, 13.99999999999999645 ) ) ;
#4703=CARTESIAN_POINT ( 'NONE',  ( 7.280083392764700179, -2.072676875633882254, 14.00000000000000000 ) ) ;
#4705=CARTESIAN_POINT ( 'NONE',  ( 7.066195124645999748, -7.302433507960749637, 1.999999999999998224 ) ) ;
#4708=CARTESIAN_POINT ( 'NONE',  ( -6.826495404309643966, 4.393449859560456083, 1.999999999999998224 ) ) ;
#4709=CARTESIAN_POINT ( 'NONE',  ( -6.112420884766618379, -2.295018720694776526, 1.999999999999998224 ) ) ;
#4710=CARTESIAN_POINT ( 'NONE',  ( 5.213743241621229707, -4.883528188333805531, 13.99999999999999645 ) ) ;
#4712=CARTESIAN_POINT ( 'NONE',  ( 1.511842404626676961, 9.183516746439465805, 1.999999999999998224 ) ) ;
#4720=CARTESIAN_POINT ( 'NONE',  ( -1.063411474431080528, -9.238278818535565762, 13.99999999999999645 ) ) ;
#4727=CARTESIAN_POINT ( 'NONE',  ( 4.415008247871436531, 7.106745273741267965, 14.00000000000000000 ) ) ;
#4728=CARTESIAN_POINT ( 'NONE',  ( -2.965071238690785371, 6.007415411094349622, 1.999999999999998224 ) ) ;
#4731=CARTESIAN_POINT ( 'NONE',  ( -2.189112655477411185, -6.464091385745795115, 14.00000000000000000 ) ) ;
#4733=CARTESIAN_POINT ( 'NONE',  ( 9.650319724628623419, 2.588775111615904567, 1.999999999999998224 ) ) ;
#4737=CARTESIAN_POINT ( 'NONE',  ( 8.518575158373787204, 0.2826087140540892162, 1.999999999999998224 ) ) ;
#4739=CARTESIAN_POINT ( 'NONE',  ( -5.432680616545222385, 3.899654942179428652, 2.000000000001176392 ) ) ;
#4740=CARTESIAN_POINT ( 'NONE',  ( 5.194219494279654015, 4.554949839096549269, 13.99999999999999645 ) ) ;
#4743=CARTESIAN_POINT ( 'NONE',  ( -0.6809175113353352904, 10.25113960786383771, 1.999999999999998224 ) ) ;
#4751=CARTESIAN_POINT ( 'NONE',  ( -6.537688394901546296, -6.759197365499824528, 13.99999999999999645 ) ) ;
#4752=FACE_OUTER_BOUND ( 'NONE', #5480, .T. ) ;
#4758=CARTESIAN_POINT ( 'NONE',  ( 7.990059919442007441, -3.149571442993018167, 14.00000000000000000 ) ) ;
#4760=CARTESIAN_POINT ( 'NONE',  ( -10.26372689808646577, -2.219791875069885290, 13.99999999999999645 ) ) ;
#4763=CARTESIAN_POINT ( 'NONE',  ( 4.064490656458173312, -6.524520197619847472, 14.00000000000000000 ) ) ;
#4765=CARTESIAN_POINT ( 'NONE',  ( 6.769338797470902946, 8.534199679356609280, 1.999999999999998224 ) ) ;
#4767=CARTESIAN_POINT ( 'NONE',  ( 0.5931392160223177834, -7.236979168992432321, 13.99999999999999645 ) ) ;
#4769=CARTESIAN_POINT ( 'NONE',  ( 8.256732931686219246, 4.597988481711511533, 1.999999999999998224 ) ) ;
#4771=CARTESIAN_POINT ( 'NONE',  ( -0.2539011084975961174, 7.766605221862830533, 1.999999999999998224 ) ) ;
#4772=CARTESIAN_POINT ( 'NONE',  ( -2.263950162103714359, 8.438937471999240714, 13.99999999999999645 ) ) ;
#4774=CARTESIAN_POINT ( 'NONE',  ( 5.071900148311750733, 7.881338450276374807, 1.999999999999998224 ) ) ;
#4779=CARTESIAN_POINT ( 'NONE',  ( 8.973806924230895987, -1.178693538871703250, 13.99999999999999645 ) ) ;
#4786=CARTESIAN_POINT ( 'NONE',  ( 6.929006764466010715, 4.804313515625074693, 14.00000000000000000 ) ) ;
#4787=CARTESIAN_POINT ( 'NONE',  ( 11.00000000000000355, -2.488243985854232676E-14, 13.99999999999999645 ) ) ;
#4789=CARTESIAN_POINT ( 'NONE',  ( 8.518575158374426692, 0.2826087140540691767, 14.00000000000000000 ) ) ;
#4793=CARTESIAN_POINT ( 'NONE',  ( 1.183015137239217696, -7.150809911821260911, 13.99999999999999645 ) ) ;
#4795=CARTESIAN_POINT ( 'NONE',  ( 2.992331685656917539, 8.840389773664522721, 1.999999999999998224 ) ) ;
#4796=CARTESIAN_POINT ( 'NONE',  ( 5.213743241621227931, -4.883528188333804643, 1.999999999999998224 ) ) ;
#4797=CARTESIAN_POINT ( 'NONE',  ( 5.862282306371745300, 6.688714470717012972, 13.99999999999999645 ) ) ;
#4804=CARTESIAN_POINT ( 'NONE',  ( -10.26372689808646577, -2.219791875069885290, 13.99999999999999645 ) ) ;
#4811=CARTESIAN_POINT ( 'NONE',  ( -0.1423371034015828429, 8.273642750286580139, 14.00000000000000000 ) ) ;
#4812=CARTESIAN_POINT ( 'NONE',  ( 1.623707939105925702, -6.078451570951504124, 1.999999999999998224 ) ) ;
#4816=CARTESIAN_POINT ( 'NONE',  ( 6.592258996018688144, -3.799026305082323418, 14.00000000000000000 ) ) ;
#4822=CARTESIAN_POINT ( 'NONE',  ( -2.466819000628047487, 6.242838961510106977, 13.99999999999999645 ) ) ;
#4824=CARTESIAN_POINT ( 'NONE',  ( 6.863489721961431478, 6.439594285167053123, 1.999999999999998224 ) ) ;
#4826=CARTESIAN_POINT ( 'NONE',  ( 0.5931392160223177834, -7.236979168992430544, 1.999999999999998224 ) ) ;
#4829=VECTOR ( 'NONE', #2909, 1000.000000000000114 ) ;
#4833=CARTESIAN_POINT ( 'NONE',  ( -2.283612537812033771, 5.775797914528922661, 1.999999999999998224 ) ) ;
#4838=CARTESIAN_POINT ( 'NONE',  ( 9.807503887221459493, -2.283819133639753751, 13.99999999999999645 ) ) ;
#4845=CARTESIAN_POINT ( 'NONE',  ( -7.425829140954380847, 3.215541426300493111, 14.00000000000000000 ) ) ;
#4846=CARTESIAN_POINT ( 'NONE',  ( -4.372214883940050534, 6.312905667202751481, 1.999999999999998224 ) ) ;
#4848=CARTESIAN_POINT ( 'NONE',  ( 6.000000000000000888, 0.000000000000000000, 7.999999999999996447 ) ) ;
#4849=CARTESIAN_POINT ( 'NONE',  ( 3.208073253695060245, -8.107602109809697311, 14.00000000000000000 ) ) ;
#4852=CARTESIAN_POINT ( 'NONE',  ( -3.867583043141952892, 8.914321633328466277, 1.999999999999998224 ) ) ;
#4853=CARTESIAN_POINT ( 'NONE',  ( -8.741731599017841248, 6.051300285686449953, 1.999999999999998224 ) ) ;
#4855=CARTESIAN_POINT ( 'NONE',  ( -6.112420884766619267, -2.295018720694776970, 13.99999999999999645 ) ) ;
#4857=CARTESIAN_POINT ( 'NONE',  ( 6.721134410589269415, -6.938257756003234356, 1.999999999999998224 ) ) ;
#4859=CARTESIAN_POINT ( 'NONE',  ( -6.505530684480364201, -3.618119970335912150, 1.999999999999998224 ) ) ;
#4863=CARTESIAN_POINT ( 'NONE',  ( 6.160418207306092242, 1.983851483784910164, 1.999999999999998224 ) ) ;
#4873=CARTESIAN_POINT ( 'NONE',  ( -1.271096247112511346, -9.720655361064800104, 14.00000000000000000 ) ) ;
#4874=CARTESIAN_POINT ( 'NONE',  ( -0.5931392160223127874, -7.263020831007572120, 1.999999999999998224 ) ) ;
#4876=CARTESIAN_POINT ( 'NONE',  ( 7.311638624438941747, 4.225618826270679307, 1.999999999999998224 ) ) ;
#4877=CARTESIAN_POINT ( 'NONE',  ( -7.550296695602809471, -2.566425989403007257, 14.00000000000000000 ) ) ;
#4879=CARTESIAN_POINT ( 'NONE',  ( -2.179108132477198367, -10.08557389312680108, 1.999999999999998224 ) ) ;
#4881=CARTESIAN_POINT ( 'NONE',  ( -1.451466707715608040, -6.203196315423898710, 13.99999999999999645 ) ) ;
#4883=CARTESIAN_POINT ( 'NONE',  ( -7.963215149404742732, -4.094909132697305054, 1.999999999999998224 ) ) ;
#4884=CARTESIAN_POINT ( 'NONE',  ( -5.322107489685658166, 5.499660323246576610, 1.999999999999998224 ) ) ;
#4885=LINE ( 'NONE', #513, #4092 ) ;
#4887=PRESENTATION_STYLE_ASSIGNMENT (( #1729 ) ) ;
#4888=CARTESIAN_POINT ( 'NONE',  ( -3.922355934210176809, -4.464780306276820099, 1.999999999999998224 ) ) ;
#4899=CARTESIAN_POINT ( 'NONE',  ( -9.926332099419621358, -1.311590842189569894, 14.00000000000000000 ) ) ;
#4900=CARTESIAN_POINT ( 'NONE',  ( -2.721086536275891810, 7.222755814214461445, 1.999999999999998224 ) ) ;
#4901=CARTESIAN_POINT ( 'NONE',  ( 3.208073253695059801, -8.107602109809695534, 1.999999999999998224 ) ) ;
#4903=CARTESIAN_POINT ( 'NONE',  ( 6.721134410589271191, -6.938257756002876420, 14.00000000000000000 ) ) ;
#4905=CARTESIAN_POINT ( 'NONE',  ( -9.197478219253614640, 5.306711421960435437, 1.999999999999998224 ) ) ;
#4908=CARTESIAN_POINT ( 'NONE',  ( 2.519353604429575011, -7.832629354751150963, 13.99999999999999645 ) ) ;
#4909=CARTESIAN_POINT ( 'NONE',  ( 7.024953159363689359, -4.052930060063556716, 13.99999999999999645 ) ) ;
#4912=CARTESIAN_POINT ( 'NONE',  ( -9.692812185270616610, 2.758747493781260829, 1.999999999999998224 ) ) ;
#4913=CARTESIAN_POINT ( 'NONE',  ( 6.679452517770526399, -4.623421500472435497, 1.999999999999998224 ) ) ;
#4914=LINE ( 'NONE', #4027, #1703 ) ;
#4919=CARTESIAN_POINT ( 'NONE',  ( 0.7175617537426045578, 6.248173425771537559, 1.999999999999998224 ) ) ;
#4922=CARTESIAN_POINT ( 'NONE',  ( 10.02932042447482353, 0.1670047327946668492, 13.99999999999999645 ) ) ;
#4929=CARTESIAN_POINT ( 'NONE',  ( 3.433597602020987072, -9.098706718024024198, 14.00000000000000000 ) ) ;
#4930=CARTESIAN_POINT ( 'NONE',  ( 0.5931392160223177834, -7.236979168992430544, 1.999999999999998224 ) ) ;
#4932=CARTESIAN_POINT ( 'NONE',  ( 5.528193227148988420, 6.314447692498917242, 1.999999999999998224 ) ) ;
#4933=CARTESIAN_POINT ( 'NONE',  ( -5.048038583874033591, -7.300734008993382318, 14.00000000000000000 ) ) ;
#4937=CARTESIAN_POINT ( 'NONE',  ( -7.044187934146015628, 6.598551529631267343, 1.999999999999998224 ) ) ;
#4939=CARTESIAN_POINT ( 'NONE',  ( -2.153669193480074018, -8.035861145135083206, 13.99999999999999645 ) ) ;
#4940=CARTESIAN_POINT ( 'NONE',  ( -5.741039858921713979, -6.128965587877692300, 13.99999999999999645 ) ) ;
#4941=CARTESIAN_POINT ( 'NONE',  ( 5.030817567586499450, 9.062633982223127660, 1.999999999999998224 ) ) ;
#4943=CARTESIAN_POINT ( 'NONE',  ( 6.401046915551857452, 6.194151307162986342, 1.999999999999998224 ) ) ;
#4945=CARTESIAN_POINT ( 'NONE',  ( 5.500000000000001776, 0.000000000000000000, 14.00000000000000000 ) ) ;
#4946=CARTESIAN_POINT ( 'NONE',  ( 5.733165789232423037, 2.946509839760266924, 1.999999999999998224 ) ) ;
#4948=ORIENTED_EDGE ( 'NONE', *, *, #3567, .F. ) ;
#4949=CARTESIAN_POINT ( 'NONE',  ( 4.290186206382708534, 5.996800006796977556, 1.999999999999998224 ) ) ;
#4957=CARTESIAN_POINT ( 'NONE',  ( -9.273719170356997665, -3.669762015051720727, 14.00000000000000000 ) ) ;
#4958=CARTESIAN_POINT ( 'NONE',  ( 6.033242055734851839, 5.122103984031729063, 1.999999999999998224 ) ) ;
#4959=CARTESIAN_POINT ( 'NONE',  ( -6.700137237869126849, -5.881230172875862472, 1.999999999999998224 ) ) ;
#4960=CARTESIAN_POINT ( 'NONE',  ( 3.713512749563263604, 8.576920285551967282, 14.00000000000000000 ) ) ;
#4962=CARTESIAN_POINT ( 'NONE',  ( 9.599547022228483328, -3.085197981542975310, 1.999999999999998224 ) ) ;
#4963=CARTESIAN_POINT ( 'NONE',  ( -2.744490807750914918, 5.556819979548927257, 14.00000000000000000 ) ) ;
#4964=CARTESIAN_POINT ( 'NONE',  ( 7.409328306158469601, 2.927536720054149555, 13.99999999999999645 ) ) ;
#4965=CARTESIAN_POINT ( 'NONE',  ( -10.03347820201762630, 0.3196629254998830660, 1.999999999999998224 ) ) ;
#4967=CARTESIAN_POINT ( 'NONE',  ( 5.933674912743041041, -6.989438080420770305, 1.999999999999998224 ) ) ;
#4969=CARTESIAN_POINT ( 'NONE',  ( -0.8169484412210608060, 6.196426872864403634, 1.999999999999998224 ) ) ;
#4971=CARTESIAN_POINT ( 'NONE',  ( -0.2403693791186040096, 7.265099133626553574, 1.999999999999998224 ) ) ;
#4978=CARTESIAN_POINT ( 'NONE',  ( -3.609299841826104416, -9.156952235374472338, 14.00000000000000000 ) ) ;
#4979=CARTESIAN_POINT ( 'NONE',  ( 2.519353604429720228, -7.832629354751149187, 1.999999999999998224 ) ) ;
#4981=CARTESIAN_POINT ( 'NONE',  ( -0.1423371034015438186, 8.273642750285960190, 1.999999999999998224 ) ) ;
#4983=CARTESIAN_POINT ( 'NONE',  ( -9.692812185271368008, 2.758747493781260385, 14.00000000000000000 ) ) ;
#4987=CARTESIAN_POINT ( 'NONE',  ( 0.7175617537426050019, 6.248173425771539335, 14.00000000000000000 ) ) ;
#4988=CARTESIAN_POINT ( 'NONE',  ( 2.810994617404221962, -9.846529629020569274, 13.99999999999999645 ) ) ;
#4990=CARTESIAN_POINT ( 'NONE',  ( -0.3669926094919908621, -5.824518274481599533, 14.00000000000000000 ) ) ;
#4993=CARTESIAN_POINT ( 'NONE',  ( -7.763712483375481810, -3.368527140560798827, 1.999999999999998224 ) ) ;
#4997=CARTESIAN_POINT ( 'NONE',  ( -1.987635485262058133, 6.951293809708865012, 1.999999999999998224 ) ) ;
#4999=CARTESIAN_POINT ( 'NONE',  ( -5.034899347481144538, -4.722558430572731503, 1.999999999999998224 ) ) ;
#5012=CARTESIAN_POINT ( 'NONE',  ( 6.452733273991772656, 8.145031704320798482, 14.00000000000000000 ) ) ;
#5013=CARTESIAN_POINT ( 'NONE',  ( -7.763712483375481810, -3.368527140560798827, 1.999999999999998224 ) ) ;
#5015=CARTESIAN_POINT ( 'NONE',  ( -9.986481889893736863, 1.144076113142370899, 1.999999999999998224 ) ) ;
#5016=CARTESIAN_POINT ( 'NONE',  ( 9.348788865899230416, 1.705571004836294646, 14.00000000000000000 ) ) ;
#5019=ORIENTED_EDGE ( 'NONE', *, *, #4034, .F. ) ;
#5020=CARTESIAN_POINT ( 'NONE',  ( 10.86297249782008123, 1.796588950249126349, 1.999999999999998224 ) ) ;
#5022=CARTESIAN_POINT ( 'NONE',  ( 1.208067634251009270, -9.180948453718622559, 13.99999999999999645 ) ) ;
#5024=CARTESIAN_POINT ( 'NONE',  ( -3.595699629853522872, 5.016010494498949868, 14.00000000000000000 ) ) ;
#5027=CARTESIAN_POINT ( 'NONE',  ( 0.5754137710878161061, 8.770917875152035137, 1.999999999999998224 ) ) ;
#5031=CARTESIAN_POINT ( 'NONE',  ( 6.523553822664517554, -0.1051741892335503609, 1.999999999999998224 ) ) ;
#5034=CARTESIAN_POINT ( 'NONE',  ( 6.592258996018686368, -3.799026305082465971, 1.999999999999998224 ) ) ;
#5040=CARTESIAN_POINT ( 'NONE',  ( 4.264126983937992499, 9.433107915010287670, 14.00000000000000000 ) ) ;
#5041=CARTESIAN_POINT ( 'NONE',  ( 0.5432484998931219611, -8.249156888542632515, 1.999999999999998224 ) ) ;
#5042=CARTESIAN_POINT ( 'NONE',  ( -6.681468852107525613, -5.130140014479350974, 13.99999999999999645 ) ) ;
#5043=CARTESIAN_POINT ( 'NONE',  ( 8.256732931686219246, 4.597988481711511533, 1.999999999999998224 ) ) ;
#5046=PRODUCT ( 'Spring Coil Unit', 'Spring Coil Unit', '', ( #4397 ) ) ;
#5047=CARTESIAN_POINT ( 'NONE',  ( 10.50003631213657762, 0.006025845833179020727, 1.999999999999998224 ) ) ;
#5050=CARTESIAN_POINT ( 'NONE',  ( -6.876639332705559937, 1.598006320995821516, 14.00000000000000000 ) ) ;
#5051=CARTESIAN_POINT ( 'NONE',  ( -0.3010823416051303103, -9.281161307073869438, 13.99999999999999645 ) ) ;
#5053=CARTESIAN_POINT ( 'NONE',  ( -6.881333183081246752, -1.254343363641206688, 14.00000000000000000 ) ) ;
#5055=CARTESIAN_POINT ( 'NONE',  ( -3.127066335681005338, 9.214240776399423183, 1.999999999999998224 ) ) ;
#5058=CARTESIAN_POINT ( 'NONE',  ( -6.881333183080980298, -1.254343363641173381, 1.999999999999998224 ) ) ;
#5060=CARTESIAN_POINT ( 'NONE',  ( 4.062840028443489793, -5.287223670286648414, 1.999999999999998224 ) ) ;
#5062=CARTESIAN_POINT ( 'NONE',  ( 6.026041665150466464, -0.9817477132364120784, 13.99999999999999645 ) ) ;
#5068=CARTESIAN_POINT ( 'NONE',  ( -2.557952627993305583, -8.967547948950716830, 1.999999999999998224 ) ) ;
#5069=CARTESIAN_POINT ( 'NONE',  ( -2.263950162103714359, 8.438937471999240714, 13.99999999999999645 ) ) ;
#5076=CARTESIAN_POINT ( 'NONE',  ( 6.680730669075651385, 3.301097878975988831, 14.00000000000000000 ) ) ;
#5078=CARTESIAN_POINT ( 'NONE',  ( 9.599547022228486881, -3.085197981543154278, 13.99999999999999645 ) ) ;
#5082=CARTESIAN_POINT ( 'NONE',  ( -0.8347742375825083494, 7.207659102801796891, 14.00000000000000000 ) ) ;
#5084=CARTESIAN_POINT ( 'NONE',  ( -8.483256258862246213, -6.077987531410204980, 1.999999999999998224 ) ) ;
#5088=CARTESIAN_POINT ( 'NONE',  ( -5.581220830680290845, 5.949058968288200688, 1.999999999999998224 ) ) ;
#5091=CARTESIAN_POINT ( 'NONE',  ( -3.231338468933299790, -7.147216519672494606, 1.999999999999998224 ) ) ;
#5092=CARTESIAN_POINT ( 'NONE',  ( 0.2194671214740537279, 6.774136816532212890, 1.999999999999998224 ) ) ;
#5093=CARTESIAN_POINT ( 'NONE',  ( 1.183015137239217696, -7.150809911821260911, 13.99999999999999645 ) ) ;
#5100=CARTESIAN_POINT ( 'NONE',  ( 0.1634456542307747284, 10.28566380800474889, 14.00000000000000000 ) ) ;
#5101=CARTESIAN_POINT ( 'NONE',  ( -5.921118896519414143, 6.318058289644735481, 1.999999999999998224 ) ) ;
#5103=CARTESIAN_POINT ( 'NONE',  ( 8.027649061864064350, -0.2602747315786822502, 13.99999999999999645 ) ) ;
#5112=CARTESIAN_POINT ( 'NONE',  ( 5.053476174606819527, -5.757900651972699180, 14.00000000000000000 ) ) ;
#5114=CARTESIAN_POINT ( 'NONE',  ( -9.247243397275783039, 2.478494142799223976, 13.99999999999999645 ) ) ;
#5115=CARTESIAN_POINT ( 'NONE',  ( 5.733165789232424814, 2.946509839760390381, 14.00000000000000000 ) ) ;
#5118=CARTESIAN_POINT ( 'NONE',  ( -9.026614039607443019, -2.903226997913650465, 1.999999999999998224 ) ) ;
#5122=CARTESIAN_POINT ( 'NONE',  ( 2.543939756934456842, 7.929199913827334356, 1.999999999999998224 ) ) ;
#5125=CARTESIAN_POINT ( 'NONE',  ( 3.909482108038855319, 5.648312977191786821, 13.99999999999999645 ) ) ;
#5133=CARTESIAN_POINT ( 'NONE',  ( -9.247243397276459831, 2.478494142799053446, 1.999999999999998224 ) ) ;
#5134=CARTESIAN_POINT ( 'NONE',  ( 9.020117466465418232, 0.2947087185667972564, 13.99999999999999645 ) ) ;
#5140=CARTESIAN_POINT ( 'NONE',  ( -6.317162512442926037, 3.238855812894408714, 14.00000000000000000 ) ) ;
#5141=CARTESIAN_POINT ( 'NONE',  ( -9.742306995815035009, -3.848972158781221786, 13.99999999999999645 ) ) ;
#5142=CARTESIAN_POINT ( 'NONE',  ( -3.597458971453999954, 6.226096630968013912, 14.00000000000000000 ) ) ;
#5144=CARTESIAN_POINT ( 'NONE',  ( -2.557952627993305583, -8.967547948950716830, 1.999999999999998224 ) ) ;
#5149=CARTESIAN_POINT ( 'NONE',  ( -3.231338468933299790, -7.147216519672494606, 1.999999999999998224 ) ) ;
#5151=CARTESIAN_POINT ( 'NONE',  ( 1.015216742983949372, 7.730330528320555672, 13.99999999999999645 ) ) ;
#5153=CARTESIAN_POINT ( 'NONE',  ( 8.172274133037948474, -5.076547540501181288, 1.999999999999998224 ) ) ;
#5157=DIRECTION ( 'NONE',  ( 0.000000000000000000, 2.258754526011467828E-18, -1.000000000000000000 ) ) ;
#5158=CARTESIAN_POINT ( 'NONE',  ( -9.406456921418632433, 1.708717176649267477, 13.99999999999999645 ) ) ;
#5159=CARTESIAN_POINT ( 'NONE',  ( -0.6809175113353355124, 10.25113960786383949, 14.00000000000000000 ) ) ;
#5160=ORIENTED_EDGE ( 'NONE', *, *, #2367, .T. ) ;
#5164=CARTESIAN_POINT ( 'NONE',  ( 7.320916985966520407, 1.587212364775818285, 14.00000000000000000 ) ) ;
#5165=CARTESIAN_POINT ( 'NONE',  ( -3.287100391418014578, 10.22059872437975869, 13.99999999999999645 ) ) ;
#5166=CARTESIAN_POINT ( 'NONE',  ( 6.445330636073146380, -1.168293168414177741, 14.00000000000000000 ) ) ;
#5168=CARTESIAN_POINT ( 'NONE',  ( 7.775655769254118610, 6.170250810330676572, 1.999999999999998224 ) ) ;
#5171=CARTESIAN_POINT ( 'NONE',  ( 7.280083392764698402, -2.072676875633882254, 1.999999999999998224 ) ) ;
#5173=CARTESIAN_POINT ( 'NONE',  ( 2.877506500681688895, 7.288437455188075731, 13.99999999999999645 ) ) ;
#5175=CARTESIAN_POINT ( 'NONE',  ( 3.433597602020624251, -9.098706718023301221, 1.999999999999998224 ) ) ;
#5176=EDGE_CURVE ( 'NONE', #2002, #3324, #5380, .T. ) ;
#5177=CARTESIAN_POINT ( 'NONE',  ( 5.500000000000001776, 0.000000000000000000, 14.00000000000000000 ) ) ;
#5185=CARTESIAN_POINT ( 'NONE',  ( -9.247243397275783039, 2.478494142799223976, 13.99999999999999645 ) ) ;
#5193=CARTESIAN_POINT ( 'NONE',  ( 1.853537052132013807, -8.546502713975392851, 14.00000000000000000 ) ) ;
#5194=CARTESIAN_POINT ( 'NONE',  ( 9.199536834907137361, 5.930433524308741156, 13.99999999999999645 ) ) ;
#5198=CARTESIAN_POINT ( 'NONE',  ( -0.1423371034015828429, 8.273642750286580139, 14.00000000000000000 ) ) ;
#5200=CARTESIAN_POINT ( 'NONE',  ( -9.197478219253614640, 5.306711421960435437, 1.999999999999998224 ) ) ;
#5202=CARTESIAN_POINT ( 'NONE',  ( -5.402835942920536816, -5.063607225391134392, 13.99999999999999645 ) ) ;
#5204=CARTESIAN_POINT ( 'NONE',  ( -3.813875884798381577, -6.869235835554530212, 1.999999999999998224 ) ) ;
#5208=CARTESIAN_POINT ( 'NONE',  ( 6.938542625487071902, -1.260128425111980643, 13.99999999999999645 ) ) ;
#5213=DIRECTION ( 'NONE',  ( 1.000000000000000000, 0.000000000000000000, 0.000000000000000000 ) ) ;
#5214=CARTESIAN_POINT ( 'NONE',  ( -7.161907081466631908, 5.673982509928833018, 1.999999999999998224 ) ) ;
#5222=CARTESIAN_POINT ( 'NONE',  ( 7.233280636258937690, 6.778630567624380099, 13.99999999999999645 ) ) ;
#5223=DIRECTION ( 'NONE',  ( 0.000000000000000000, 0.000000000000000000, -1.000000000000000000 ) ) ;
#5228=CARTESIAN_POINT ( 'NONE',  ( -5.081985621531964981, 6.397721742171718518, 14.00000000000000000 ) ) ;
#5229=CARTESIAN_POINT ( 'NONE',  ( 3.909482108038854431, 5.648312977191785045, 1.999999999999998224 ) ) ;
#5232=CARTESIAN_POINT ( 'NONE',  ( 0.5385325299235224072, 8.270587056550175120, 14.00000000000000000 ) ) ;
#5236=CARTESIAN_POINT ( 'NONE',  ( 4.366464973618273682, -5.686602709308030690, 13.99999999999999645 ) ) ;
#5238=CARTESIAN_POINT ( 'NONE',  ( -5.592500163775054212, 7.275211197852026856, 1.999999999999998224 ) ) ;
#5239=CARTESIAN_POINT ( 'NONE',  ( 4.366464973618271905, -5.686602709308029802, 1.999999999999998224 ) ) ;
#5240=CARTESIAN_POINT ( 'NONE',  ( -8.513020831365363250, 0.6954046021538080602, 13.99999999999999645 ) ) ;
#5244=PLANE ( 'NONE',  #2077 ) ;
#5248=CARTESIAN_POINT ( 'NONE',  ( 8.993528569561179964, -4.616306094804236260, 13.99999999999999645 ) ) ;
#5254=CARTESIAN_POINT ( 'NONE',  ( -6.667513054348625623, -4.302816426345352774, 14.00000000000000000 ) ) ;
#5255=CARTESIAN_POINT ( 'NONE',  ( -6.045729098460493667, -8.441868823237593134, 13.99999999999999645 ) ) ;
#5257=CARTESIAN_POINT ( 'NONE',  ( 3.857245400775171529, -7.804869966781184054, 14.00000000000000000 ) ) ;
#5262=CARTESIAN_POINT ( 'NONE',  ( -5.978927507574435474, 2.933119789328458182, 13.99999999999999645 ) ) ;
#5263=CARTESIAN_POINT ( 'NONE',  ( -8.757712506721389900, -2.046213373001789737, 1.999999999999998224 ) ) ;
#5264=CARTESIAN_POINT ( 'NONE',  ( -3.845892476879857025, 6.661954734853423155, 1.999999999999998224 ) ) ;
#5269=CARTESIAN_POINT ( 'NONE',  ( 5.500000000000000000, 0.000000000000000000, 1.999999999999998224 ) ) ;
#5280=CARTESIAN_POINT ( 'NONE',  ( 6.037635170864974477, 5.848285684831325604, 14.00000000000000000 ) ) ;
#5281=CARTESIAN_POINT ( 'NONE',  ( -7.364573508975982286, 1.714675912027187943, 1.999999999999998224 ) ) ;
#5285=CARTESIAN_POINT ( 'NONE',  ( 5.612687125618119666, -6.603876269260188892, 14.00000000000000000 ) ) ;
#5288=CARTESIAN_POINT ( 'NONE',  ( -7.551678268146208239, 5.989845445213456188, 1.999999999999998224 ) ) ;
#5290=CARTESIAN_POINT ( 'NONE',  ( -2.352725117874390648, -6.938351456669185069, 13.99999999999999645 ) ) ;
#5292=CARTESIAN_POINT ( 'NONE',  ( 5.071900148311750733, 7.881338450276374807, 1.999999999999998224 ) ) ;
#5293=CARTESIAN_POINT ( 'NONE',  ( 6.180183843827202317, 3.174252413088801461, 1.999999999999998224 ) ) ;
#5296=CARTESIAN_POINT ( 'NONE',  ( 5.526041665711819206, -0.8982374663919266977, 1.999999999999998224 ) ) ;
#5303=CARTESIAN_POINT ( 'NONE',  ( 10.02239396097876423, -0.6576683464575836524, 13.99999999999999645 ) ) ;
#5309=CARTESIAN_POINT ( 'NONE',  ( -5.048038583874033591, -7.300734008993382318, 14.00000000000000000 ) ) ;
#5310=CARTESIAN_POINT ( 'NONE',  ( 6.209839678910233474, -3.451293940533043614, 1.999999999999998224 ) ) ;
#5313=CARTESIAN_POINT ( 'NONE',  ( -1.390902631672706224, -7.679604985168660747, 14.00000000000000000 ) ) ;
#5316=CARTESIAN_POINT ( 'NONE',  ( -10.26372689808571970, -2.219791875069699216, 1.999999999999998224 ) ) ;
#5317=CARTESIAN_POINT ( 'NONE',  ( 8.671201137383034663, 6.657490096169006222, 1.999999999999998224 ) ) ;
#5318=CARTESIAN_POINT ( 'NONE',  ( -2.919577271296576182, -6.733962781534541975, 13.99999999999999645 ) ) ;
#5320=CARTESIAN_POINT ( 'NONE',  ( 1.124407659250306279, -9.699258357302506184, 1.999999999999998224 ) ) ;
#5321=CARTESIAN_POINT ( 'NONE',  ( -2.352725117874390204, -6.938351456669183293, 1.999999999999998224 ) ) ;
#5324=CARTESIAN_POINT ( 'NONE',  ( 10.36702220812592223, 1.720931399333113676, 1.999999999999998224 ) ) ;
#5335=CARTESIAN_POINT ( 'NONE',  ( -2.970508497641844325, 8.737606122599315128, 14.00000000000000000 ) ) ;
#5336=CARTESIAN_POINT ( 'NONE',  ( -6.505530684480364201, -3.618119970335912150, 1.999999999999998224 ) ) ;
#5337=CARTESIAN_POINT ( 'NONE',  ( 8.370269057507494281, -1.803949267857694716, 1.999999999999998224 ) ) ;
#5338=CARTESIAN_POINT ( 'NONE',  ( 5.519166806814065573, -7.959527472086049826, 14.00000000000000000 ) ) ;
#5340=CARTESIAN_POINT ( 'NONE',  ( -10.17357856257854110, 2.902115915870757679, 1.999999999999998224 ) ) ;
#5341=CARTESIAN_POINT ( 'NONE',  ( -0.3669926094919908621, -5.824518274481599533, 14.00000000000000000 ) ) ;
#5342=CARTESIAN_POINT ( 'NONE',  ( 6.033242055734853615, 5.122103984031451063, 13.99999999999999645 ) ) ;
#5343=CARTESIAN_POINT ( 'NONE',  ( -0.8890388043606451962, 7.706404363472290520, 13.99999999999999645 ) ) ;
#5344=CARTESIAN_POINT ( 'NONE',  ( -7.161907081466631908, 5.673982509928833018, 1.999999999999998224 ) ) ;
#5346=CARTESIAN_POINT ( 'NONE',  ( 8.640499015841685448, 2.466831329604985079, 1.999999999999998224 ) ) ;
#5349=( NAMED_UNIT ( * ) PLANE_ANGLE_UNIT ( ) SI_UNIT ( $, .RADIAN. ) );
#5351=CARTESIAN_POINT ( 'NONE',  ( -0.8169484412210608060, 6.196426872864403634, 1.999999999999998224 ) ) ;
#5355=CARTESIAN_POINT ( 'NONE',  ( -4.892757975385814362, 9.527326283048992650, 13.99999999999999645 ) ) ;
#5362=CARTESIAN_POINT ( 'NONE',  ( 1.511842404626676961, 9.183516746439467582, 14.00000000000000000 ) ) ;
#5363=CARTESIAN_POINT ( 'NONE',  ( 6.679452517770526399, -4.623421500472435497, 1.999999999999998224 ) ) ;
#5365=CARTESIAN_POINT ( 'NONE',  ( 1.147089839255700294, -8.682979827541576157, 1.999999999999998224 ) ) ;
#5366=CARTESIAN_POINT ( 'NONE',  ( 2.678407690932720353, -9.362678857628843332, 14.00000000000000000 ) ) ;
#5368=CARTESIAN_POINT ( 'NONE',  ( 5.348203032363056053, 8.300083771889280371, 1.999999999999998224 ) ) ;
#5371=CARTESIAN_POINT ( 'NONE',  ( 8.640499015841685448, 2.466831329604985079, 13.99999999999999645 ) ) ;
#5373=CARTESIAN_POINT ( 'NONE',  ( -8.440272934376814362, 1.393994921405934173, 13.99999999999999645 ) ) ;
#5375=CARTESIAN_POINT ( 'NONE',  ( -5.525185448606695360, 2.707100724334913444, 14.00000000000000000 ) ) ;
#5377=CARTESIAN_POINT ( 'NONE',  ( 8.859712399100347469, -1.914114158827000312, 1.999999999999998224 ) ) ;
#5380=LINE ( 'NONE', #4945, #2895 ) ;
#5381=CARTESIAN_POINT ( 'NONE',  ( 0.7175617537426045578, 6.248173425771537559, 1.999999999999998224 ) ) ;
#5386=CARTESIAN_POINT ( 'NONE',  ( -5.623512120026317618, -3.262381593763366450, 13.99999999999999645 ) ) ;
#5393=CARTESIAN_POINT ( 'NONE',  ( -4.983290658054754019, 7.721050520723660604, 14.00000000000000000 ) ) ;
#5394=CARTESIAN_POINT ( 'NONE',  ( 6.938542625487070126, -1.260128425111949557, 1.999999999999998224 ) ) ;
#5395=CARTESIAN_POINT ( 'NONE',  ( 2.543939756934456842, 7.929199913827334356, 1.999999999999998224 ) ) ;
#5396=CARTESIAN_POINT ( 'NONE',  ( -9.273719170356997665, -3.669762015051720727, 14.00000000000000000 ) ) ;
#5399=CARTESIAN_POINT ( 'NONE',  ( 8.993528569561179964, -4.616306094804414784, 1.999999999999998224 ) ) ;
#5400=CARTESIAN_POINT ( 'NONE',  ( -5.637968025906140213, -2.116521738900702942, 14.00000000000000000 ) ) ;
#5401=CARTESIAN_POINT ( 'NONE',  ( 4.043470907200354070, 7.877814422642792636, 13.99999999999999645 ) ) ;
#5403=CARTESIAN_POINT ( 'NONE',  ( 1.730265954310492571, 6.073542049876724747, 14.00000000000000000 ) ) ;
#5405=CARTESIAN_POINT ( 'NONE',  ( -8.388197440586290909, -1.387539741535495974, 1.999999999999998224 ) ) ;
#5408=CARTESIAN_POINT ( 'NONE',  ( 3.173694703385744997, 5.505084763670540227, 1.999999999999998224 ) ) ;
#5409=ORIENTED_EDGE ( 'NONE', *, *, #3580, .F. ) ;
#5410=CARTESIAN_POINT ( 'NONE',  ( 7.320916985966518631, 1.587212364775676843, 1.999999999999998224 ) ) ;
#5419=CARTESIAN_POINT ( 'NONE',  ( -7.559400777704423646, -6.425066744314204215, 14.00000000000000000 ) ) ;
#5420=CARTESIAN_POINT ( 'NONE',  ( -7.091148812992122963, -4.571561645352110403, 1.999999999999998224 ) ) ;
#5421=CARTESIAN_POINT ( 'NONE',  ( 7.990059919442647818, -3.149571442993177595, 1.999999999999998224 ) ) ;
#5422=CARTESIAN_POINT ( 'NONE',  ( -1.515482495401828000, 9.129776367295956874, 14.00000000000000000 ) ) ;
#5426=CARTESIAN_POINT ( 'NONE',  ( -3.987231204388229422, 4.693390172674912542, 13.99999999999953104 ) ) ;
#5427=CARTESIAN_POINT ( 'NONE',  ( 1.870926337630180569, -8.025887876971657064, 13.99999999999999645 ) ) ;
#5429=CARTESIAN_POINT ( 'NONE',  ( -9.273719170356997665, -3.669762015052091098, 1.999999999999998224 ) ) ;
#5431=CARTESIAN_POINT ( 'NONE',  ( -4.060726170632605658, -7.305992298388374273, 1.999999999999998224 ) ) ;
#5433=CARTESIAN_POINT ( 'NONE',  ( -2.547213823411294431, 6.752160688201485073, 1.999999999999998224 ) ) ;
#5435=CARTESIAN_POINT ( 'NONE',  ( 2.161943361801394570, -6.363123982928429179, 1.999999999999998224 ) ) ;
#5437=CARTESIAN_POINT ( 'NONE',  ( 6.000000000000001776, 0.000000000000000000, 13.99999999999999645 ) ) ;
#5445=CARTESIAN_POINT ( 'NONE',  ( -4.060726170632605658, -7.305992298388374273, 1.999999999999998224 ) ) ;
#5446=CARTESIAN_POINT ( 'NONE',  ( 9.527640065893086430, 0.1642265212908741445, 1.999999999999998224 ) ) ;
#5448=CARTESIAN_POINT ( 'NONE',  ( -8.913799778910966864, 1.613954699392568859, 14.00000000000000000 ) ) ;
#5453=CARTESIAN_POINT ( 'NONE',  ( -4.581738566658776435, -9.288989786611782762, 13.99999999999999645 ) ) ;
#5455=CARTESIAN_POINT ( 'NONE',  ( 10.48651993945612126, 0.8648464362367445091, 1.999999999999998224 ) ) ;
#5458=CARTESIAN_POINT ( 'NONE',  ( -5.210352092881994857, -6.569156856910357334, 1.999999999999998224 ) ) ;
#5459=AXIS2_PLACEMENT_3D ( 'NONE', #4848, #2576, #469 ) ;
#5462=CARTESIAN_POINT ( 'NONE',  ( -6.048456868091350636, 0.8014113234715940504, 1.999999999999998224 ) ) ;
#5465=CARTESIAN_POINT ( 'NONE',  ( -2.547213823411294431, 6.752160688201485073, 1.999999999999998224 ) ) ;
#5475=CARTESIAN_POINT ( 'NONE',  ( 1.870926337630253622, -8.025887876971653512, 1.999999999999998224 ) ) ;
#5476=CARTESIAN_POINT ( 'NONE',  ( 1.870926337630180569, -8.025887876971657064, 13.99999999999999645 ) ) ;
#5478=CARTESIAN_POINT ( 'NONE',  ( -3.139313036748680563, 9.741172307226465321, 1.999999999999998224 ) ) ;
#5480=EDGE_LOOP ( 'NONE', ( #4948, #2658, #427, #5019 ) ) ;
#5484=CARTESIAN_POINT ( 'NONE',  ( -7.019001384594682591, 0.4577903460187995877, 14.00000000000000000 ) ) ;
#5485=CARTESIAN_POINT ( 'NONE',  ( -3.127066335681350395, 9.214240776398044730, 13.99999999999999645 ) ) ;
#5487=CARTESIAN_POINT ( 'NONE',  ( 6.452733273992156349, 8.145031704320794930, 1.999999999999998224 ) ) ;
#5490=CARTESIAN_POINT ( 'NONE',  ( 5.099673838352487998, -8.834479793761566668, 1.999999999999998224 ) ) ;
#5493=CARTESIAN_POINT ( 'NONE',  ( 5.772253124442284111, -3.205917188174072230, 1.999999999999998224 ) ) ;
#5496=CARTESIAN_POINT ( 'NONE',  ( 2.369394374793902802, -7.353877281245869035, 1.999999999999998224 ) ) ;
#5505=CARTESIAN_POINT ( 'NONE',  ( 2.667884741302309681, 9.975564253400266423, 14.00000000000000000 ) ) ;
#5506=CARTESIAN_POINT ( 'NONE',  ( -4.227552200850895225, 7.601683304540809871, 1.999999999999998224 ) ) ;
#5507=CARTESIAN_POINT ( 'NONE',  ( 7.812003909081977504, 1.689803927524662797, 13.99999999999999645 ) ) ;
#5513=CARTESIAN_POINT ( 'NONE',  ( 4.062840028443491569, -5.287223670286397059, 14.00000000000000000 ) ) ;
#5514=CARTESIAN_POINT ( 'NONE',  ( 9.807503887221459493, -2.283819133639753751, 13.99999999999999645 ) ) ;
#5515=CARTESIAN_POINT ( 'NONE',  ( -6.065725208710916583, -3.376743199310593635, 14.00000000000000000 ) ) ;
#5517=CARTESIAN_POINT ( 'NONE',  ( -8.745075223330342595, 3.959260399367897421, 1.999999999999998224 ) ) ;
#5520=CARTESIAN_POINT ( 'NONE',  ( 6.941605245898607279, 2.746080019686067519, 1.999999999999998224 ) ) ;
#5522=CARTESIAN_POINT ( 'NONE',  ( 0.9466184546083533657, 7.233353930637701268, 1.999999999999998224 ) ) ;
#5523=CARTESIAN_POINT ( 'NONE',  ( 1.623707939105925702, -6.078451570951504124, 1.999999999999998224 ) ) ;
#5524=CARTESIAN_POINT ( 'NONE',  ( -6.465640026559317022, 4.020973141382162552, 13.99999999999999645 ) ) ;
#5526=EDGE_CURVE ( 'NONE', #3324, #261, #2475, .T. ) ;
#5531=CARTESIAN_POINT ( 'NONE',  ( 9.925004466819306259, 3.374327561486830440, 14.00000000000000000 ) ) ;
#5532=CARTESIAN_POINT ( 'NONE',  ( -8.126042061586874254, 2.755650963504471473, 1.999999999999998224 ) ) ;
#5534=CARTESIAN_POINT ( 'NONE',  ( 7.761517335261691741, -2.213789340049631349, 13.99999999999999645 ) ) ;
#5541=CARTESIAN_POINT ( 'NONE',  ( 3.247347166530789586, 6.590896817052466439, 14.00000000000000000 ) ) ;
#5542=CARTESIAN_POINT ( 'NONE',  ( 5.933674912743042817, -6.989438080420771193, 13.99999999999999645 ) ) ;
#5543=CARTESIAN_POINT ( 'NONE',  ( -7.019651866616807290, -0.1200674265790614287, 14.00000000000000000 ) ) ;
#5545=CARTESIAN_POINT ( 'NONE',  ( 8.697835924490032511, 4.836984431370230375, 1.999999999999998224 ) ) ;
#5550=CARTESIAN_POINT ( 'NONE',  ( 0.5385325299235221852, 8.270587056550796845, 1.999999999999998224 ) ) ;
#5552=CARTESIAN_POINT ( 'NONE',  ( 1.869626052002640648, 6.555486721476421863, 13.99999999999999645 ) ) ;
#5555=DIRECTION ( 'NONE',  ( 1.000000000000000000, 0.000000000000000000, 0.000000000000000000 ) ) ;
#5560=CARTESIAN_POINT ( 'NONE',  ( -9.500632974892678106, -0.6255030753161154866, 1.999999999999998224 ) ) ;
#5562=CARTESIAN_POINT ( 'NONE',  ( -9.026614039607444795, -2.903226997913483487, 13.99999999999999645 ) ) ;
#5563=CARTESIAN_POINT ( 'NONE',  ( -6.708753103182797162, 7.642576097240647570, 14.00000000000000000 ) ) ;
#5569=CARTESIAN_POINT ( 'NONE',  ( -7.019651866616807290, -0.1200674265790614287, 14.00000000000000000 ) ) ;
#5570=CARTESIAN_POINT ( 'NONE',  ( 3.605080641953931853, -9.570177220922108319, 13.99999999999999645 ) ) ;
#5572=CARTESIAN_POINT ( 'NONE',  ( 3.621982275015807939, -5.614208739972780471, 14.00000000000000000 ) ) ;
#5575=CARTESIAN_POINT ( 'NONE',  ( 0.7976699882155456889, 9.763020831628287155, 1.999999999999998224 ) ) ;
#5579=CARTESIAN_POINT ( 'NONE',  ( 4.776808680784692562, 5.634249062854761014, 1.999999999999998224 ) ) ;
#5580=CARTESIAN_POINT ( 'NONE',  ( -1.451466707715830973, -6.203196315423896934, 1.999999999999998224 ) ) ;
#5582=CARTESIAN_POINT ( 'NONE',  ( -7.211577653563209900, 2.317451195016654975, 13.99999999999999645 ) ) ;
#5583=CARTESIAN_POINT ( 'NONE',  ( 9.123540010895986541, -2.926742269086382908, 1.999999999999998224 ) ) ;
#5591=CARTESIAN_POINT ( 'NONE',  ( -5.337360893036674270, -7.710592058383929803, 13.99999999999999645 ) ) ;
#5592=CARTESIAN_POINT ( 'NONE',  ( 7.108868828250529681, 7.597268273415099138, 14.00000000000000000 ) ) ;
#5597=CARTESIAN_POINT ( 'NONE',  ( -3.597458971453999954, 6.226096630968013912, 14.00000000000000000 ) ) ;
#5598=CARTESIAN_POINT ( 'NONE',  ( -5.623512120026769701, -3.262381593762911258, 1.999999999999998224 ) ) ;
#5600=CARTESIAN_POINT ( 'NONE',  ( 5.648567055624232225, 4.800053419556652656, 14.00000000000000000 ) ) ;
#5602=CARTESIAN_POINT ( 'NONE',  ( 1.176163838800080574, -10.19826953922189539, 1.999999999999998224 ) ) ;
#5605=CARTESIAN_POINT ( 'NONE',  ( 7.311638624438941747, 4.225618826270679307, 1.999999999999998224 ) ) ;
#5606=CARTESIAN_POINT ( 'NONE',  ( -3.379911625893426308, -5.460782782531098611, 1.999999999999998224 ) ) ;
#5607=CARTESIAN_POINT ( 'NONE',  ( -5.810612947750823487, -4.611264106266947493, 13.99999999999999645 ) ) ;
#5608=CARTESIAN_POINT ( 'NONE',  ( -9.445900372709948201, 3.550092993115765871, 1.999999999999998224 ) ) ;
#5615=CARTESIAN_POINT ( 'NONE',  ( 8.859712399101631775, -1.914114158827161294, 13.99999999999999645 ) ) ;
#5621=CARTESIAN_POINT ( 'NONE',  ( 8.477027301005275461, -1.108685663976147318, 14.00000000000000000 ) ) ;
#5622=CARTESIAN_POINT ( 'NONE',  ( 2.803319092186594474, 10.45862564946370021, 13.99999999999999645 ) ) ;
#5625=CARTESIAN_POINT ( 'NONE',  ( -5.395431796987672612, -5.765308706272596950, 14.00000000000000000 ) ) ;
#5633=CARTESIAN_POINT ( 'NONE',  ( 0.5141566911143078400, -7.748312628312726602, 1.999999999999998224 ) ) ;
#5635=CARTESIAN_POINT ( 'NONE',  ( -7.227555219266157849, -1.939125212622549999, 13.99999999999999645 ) ) ;
#5636=CARTESIAN_POINT ( 'NONE',  ( 5.030817567586499450, 9.062633982223127660, 1.999999999999998224 ) ) ;
#5645=CARTESIAN_POINT ( 'NONE',  ( 0.5754137710878940437, 8.770917875152660415, 13.99999999999999645 ) ) ;
#5653=CARTESIAN_POINT ( 'NONE',  ( -2.138212235155100061, 7.953261502403491612, 14.00000000000000000 ) ) ;
#5654=CARTESIAN_POINT ( 'NONE',  ( -2.466819000628106551, 6.242838961510105200, 1.999999999999998224 ) ) ;
#5657=CARTESIAN_POINT ( 'NONE',  ( 8.156937663706065322, 2.333191796391004047, 14.00000000000000000 ) ) ;
#5661=CARTESIAN_POINT ( 'NONE',  ( -6.505530684480628878, -3.618119970335913038, 13.99999999999999645 ) ) ;
#5663=CARTESIAN_POINT ( 'NONE',  ( -0.2798806129216870886, -8.779921314118375619, 1.999999999999998224 ) ) ;
#5665=CARTESIAN_POINT ( 'NONE',  ( -1.189470317277863121, -7.202885406307536265, 1.999999999999998224 ) ) ;
#5666=CARTESIAN_POINT ( 'NONE',  ( -0.1359230501496729582, -8.279147739301068398, 13.99999999999999645 ) ) ;
#5670=DIRECTION ( 'NONE',  ( 0.000000000000000000, 0.000000000000000000, 1.000000000000000000 ) ) ;
#5674=CARTESIAN_POINT ( 'NONE',  ( -8.017392084630589721, -4.988806607527435766, 13.99999999999999645 ) ) ;
#5682=CARTESIAN_POINT ( 'NONE',  ( -4.424777426322135554, -7.679192617324877901, 14.00000000000000000 ) ) ;
#5683=CARTESIAN_POINT ( 'NONE',  ( -10.48421140591525713, 1.206973991593908169, 13.99999999999999645 ) ) ;
#5685=CARTESIAN_POINT ( 'NONE',  ( 6.591354251721611490, -5.587324598951901145, 14.00000000000000000 ) ) ;
#5717=COLOUR_RGB('Grey',0.48,0.52,0.57);
#5718=FILL_AREA_STYLE_COLOUR('',#5717);
#5719=FILL_AREA_STYLE('',(#5718));
#5720=SURFACE_STYLE_FILL_AREA(#5719);
#5721=SURFACE_SIDE_STYLE('',(#5720));
#5722=SURFACE_STYLE_USAGE(.BOTH.,#5721);
#5723=PRESENTATION_STYLE_ASSIGNMENT((#5722));
ENDSEC;
END-ISO-10303-21;
